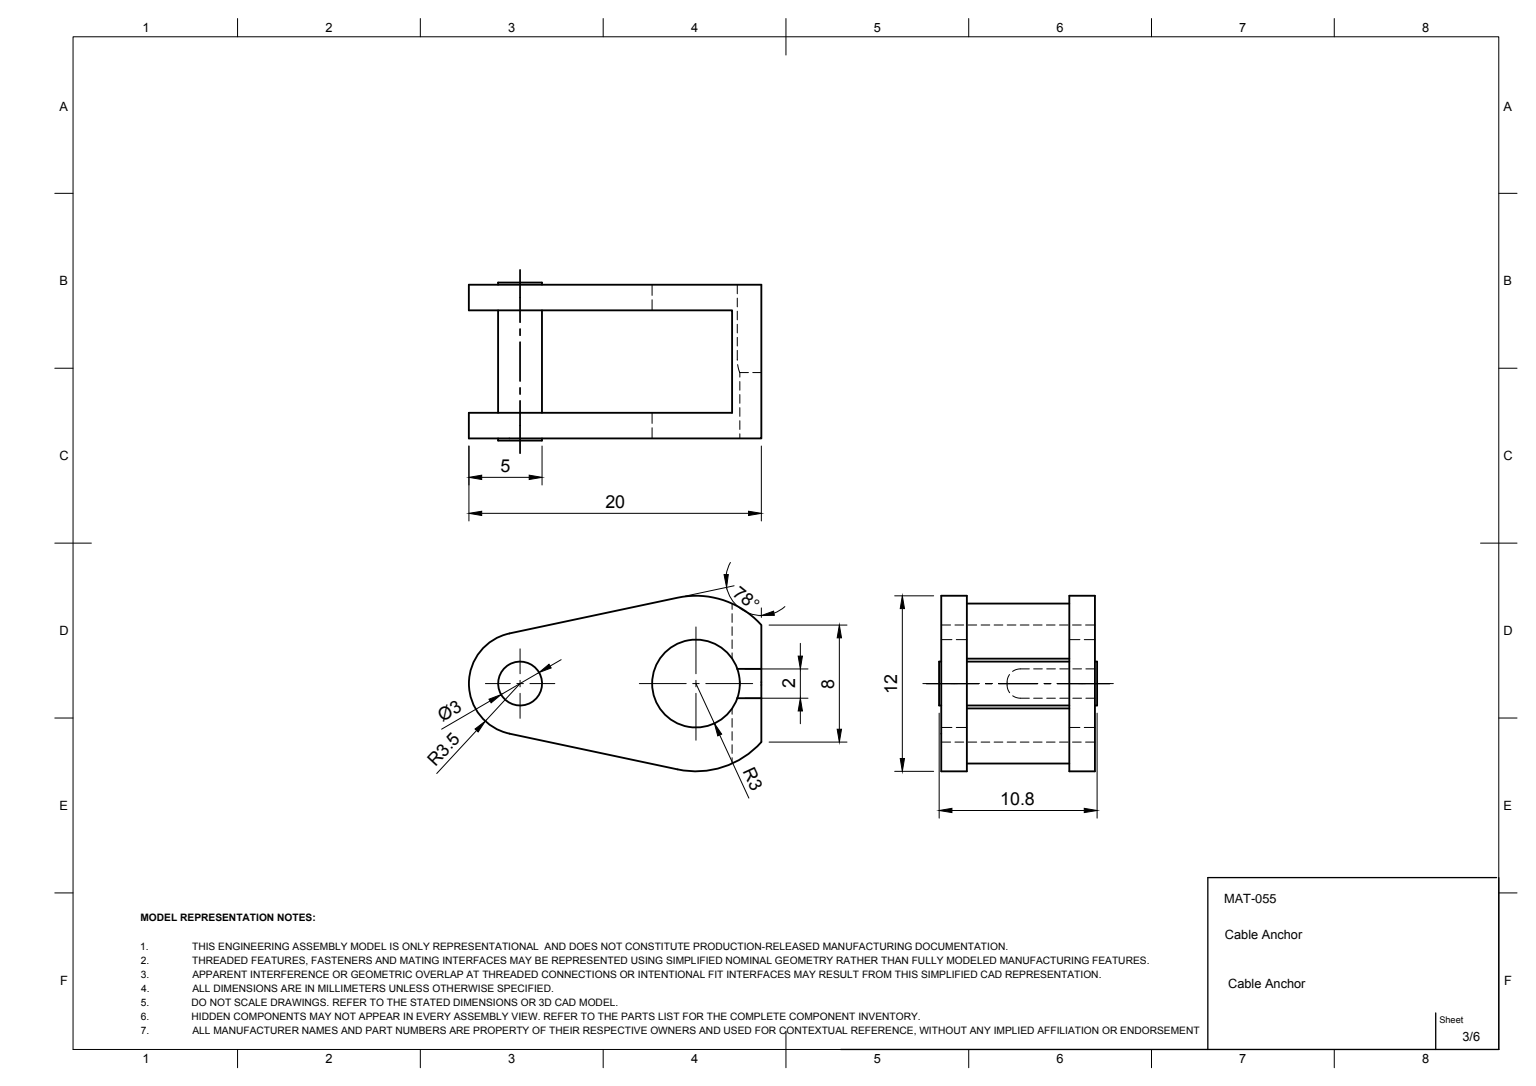
ISO-10303-21;
HEADER;
FILE_DESCRIPTION (('STEP AP214'),
    '1' );
FILE_NAME ('Cable Anchor.step',
    '2026-10-30T09:41:00',
    ( '' ),
    ( '' ),
    'SwSTEP 2.0',
    'SolidWorks 2020',
    '' );
FILE_SCHEMA (( 'AUTOMOTIVE_DESIGN' ));
ENDSEC;

DATA;
#81=ORIENTED_EDGE ( 'NONE', *, *, #25738, .F. ) ;
#83=CARTESIAN_POINT ( 'NONE',  ( 86.34560043013698305, -9.320000780048239619, -16.89321520033831447 ) ) ;
#175=AXIS2_PLACEMENT_3D ( 'NONE', #36006, #42871, #25989 ) ;
#203=EDGE_CURVE ( 'NONE', #36947, #44995, #9172, .T. ) ;
#218=CARTESIAN_POINT ( 'NONE',  ( 89.13600071704317429, -10.42165226880396567, -14.07015947738872796 ) ) ;
#224=LINE ( 'NONE', #17347, #39403 ) ;
#244=EDGE_LOOP ( 'NONE', ( #3351, #8690, #1510, #25931, #38519, #27404, #20407, #392, #9598, #8626 ) ) ;
#260=VECTOR ( 'NONE', #38746, 1000.000000000000000 ) ;
#392=ORIENTED_EDGE ( 'NONE', *, *, #6669, .F. ) ;
#446=CYLINDRICAL_SURFACE ( 'NONE', #37941, 1.499999999999996225 ) ;
#523=VERTEX_POINT ( 'NONE', #21002 ) ;
#586=LINE ( 'NONE', #7416, #43252 ) ;
#637=CARTESIAN_POINT ( 'NONE',  ( 77.25325688895158294, -4.012910213732562070, -16.89321520033831447 ) ) ;
#742=ORIENTED_EDGE ( 'NONE', *, *, #32280, .T. ) ;
#831=PRODUCT_DEFINITION_SHAPE ( 'NONE', 'NONE',  #16477 ) ;
#848=LINE ( 'NONE', #18639, #17728 ) ;
#855=DIRECTION ( 'NONE',  ( 0.000000000000000000, 0.000000000000000000, -1.000000000000000000 ) ) ;
#861=EDGE_CURVE ( 'NONE', #37401, #29422, #44018, .T. ) ;
#882=LINE ( 'NONE', #14801, #2318 ) ;
#1093=DIRECTION ( 'NONE',  ( 0.5040994586965589219, 0.8636456077245089347, 0.000000000000000000 ) ) ;
#1108=ORIENTED_EDGE ( 'NONE', *, *, #40951, .T. ) ;
#1150=DIRECTION ( 'NONE',  ( 0.5040994586965589219, 0.8636456077245089347, 0.000000000000000000 ) ) ;
#1340=CARTESIAN_POINT ( 'NONE',  ( 88.41031260927115909, -11.49916342651943957, -13.77494911842194369 ) ) ;
#1447=CARTESIAN_POINT ( 'NONE',  ( 83.75466360696344736, -7.807702403958562520, -8.143215200338314474 ) ) ;
#1510=ORIENTED_EDGE ( 'NONE', *, *, #22776, .F. ) ;
#1585=VECTOR ( 'NONE', #34649, 1000.000000000000000 ) ;
#1711=ORIENTED_EDGE ( 'NONE', *, *, #19855, .F. ) ;
#1718=CARTESIAN_POINT ( 'NONE',  ( 85.72471707980444933, -15.28778963902104060, -16.89321520033831447 ) ) ;
#1721=LINE ( 'NONE', #29548, #15713 ) ;
#1789=DIRECTION ( 'NONE',  ( 0.000000000000000000, 0.000000000000000000, 1.000000000000000000 ) ) ;
#1790=CARTESIAN_POINT ( 'NONE',  ( 82.31000308962319423, -13.76004065658516673, -8.143215200338314474 ) ) ;
#1794=CARTESIAN_POINT ( 'NONE',  ( 89.29245855188943892, -9.882163754870950001, -18.64321520033831803 ) ) ;
#1818=ORIENTED_EDGE ( 'NONE', *, *, #22126, .F. ) ;
#1835=CARTESIAN_POINT ( 'NONE',  ( 86.34560043013698305, -9.320000780048239619, -16.89321520033831447 ) ) ;
#1843=AXIS2_PLACEMENT_3D ( 'NONE', #8029, #11011, #28565 ) ;
#1857=PLANE ( 'NONE',  #19264 ) ;
#1947=DIRECTION ( 'NONE',  ( 0.6725995567522981000, 0.7400066460894877407, -0.000000000000000000 ) ) ;
#2013=EDGE_LOOP ( 'NONE', ( #16435, #12122, #81, #28622 ) ) ;
#2022=AXIS2_PLACEMENT_3D ( 'NONE', #28422, #15182, #21574 ) ;
#2037=EDGE_CURVE ( 'NONE', #38611, #14451, #22949, .T. ) ;
#2041=APPLICATION_CONTEXT ( 'automotive_design' ) ;
#2123=ORIENTED_EDGE ( 'NONE', *, *, #31988, .T. ) ;
#2144=DIRECTION ( 'NONE',  ( 0.8636456077245086016, -0.5040994586965593660, 0.000000000000000000 ) ) ;
#2184=EDGE_CURVE ( 'NONE', #38164, #19850, #25845, .T. ) ;
#2190=AXIS2_PLACEMENT_3D ( 'NONE', #12234, #8583, #22482 ) ;
#2195=VECTOR ( 'NONE', #28078, 1000.000000000000000 ) ;
#2318=VECTOR ( 'NONE', #7951, 1000.000000000000000 ) ;
#2389=DIRECTION ( 'NONE',  ( 0.000000000000000000, 0.000000000000000000, -1.000000000000000000 ) ) ;
#2435=CIRCLE ( 'NONE', #27952, 3.000000000000003997 ) ;
#2479=LINE ( 'NONE', #40116, #8942 ) ;
#2562=ORIENTED_EDGE ( 'NONE', *, *, #42601, .F. ) ;
#2639=PRODUCT_CONTEXT ( 'NONE', #2041, 'mechanical' ) ;
#2753=DIRECTION ( 'NONE',  ( -0.8636456077245080465, 0.5040994586965603652, 0.000000000000000000 ) ) ;
#2819=DIRECTION ( 'NONE',  ( 0.000000000000000000, 0.000000000000000000, 1.000000000000000000 ) ) ;
#2828=CARTESIAN_POINT ( 'NONE',  ( 89.70384154612264638, -12.43804770190545561, -13.24321520033830879 ) ) ;
#2894=ADVANCED_FACE ( 'NONE', ( #41375 ), #10569, .T. ) ;
#2910=ORIENTED_EDGE ( 'NONE', *, *, #16133, .T. ) ;
#2921=CIRCLE ( 'NONE', #20410, 1.499999999999996225 ) ;
#2971=CARTESIAN_POINT ( 'NONE',  ( 89.28655680551213436, -9.912712791071484730, -13.47323746212486562 ) ) ;
#2980=CYLINDRICAL_SURFACE ( 'NONE', #7519, 1.499999999999996225 ) ;
#2984=CIRCLE ( 'NONE', #11775, 3.000000000000003997 ) ;
#3002=ADVANCED_FACE ( 'NONE', ( #31747 ), #25144, .T. ) ;
#3083=CARTESIAN_POINT ( 'NONE',  ( 77.25325688895158294, -4.012910213732562070, -18.79321520033831661 ) ) ;
#3163=ORIENTED_EDGE ( 'NONE', *, *, #17306, .F. ) ;
#3280=VECTOR ( 'NONE', #28746, 1000.000000000000000 ) ;
#3313=EDGE_CURVE ( 'NONE', #6780, #34510, #28571, .T. ) ;
#3351=ORIENTED_EDGE ( 'NONE', *, *, #7188, .F. ) ;
#3382=EDGE_CURVE ( 'NONE', #44507, #41378, #20454, .T. ) ;
#3438=ORIENTED_EDGE ( 'NONE', *, *, #4563, .T. ) ;
#3451=( GEOMETRIC_REPRESENTATION_CONTEXT ( 3 ) GLOBAL_UNCERTAINTY_ASSIGNED_CONTEXT ( ( #12242 ) ) GLOBAL_UNIT_ASSIGNED_CONTEXT ( ( #15675, #12263, #22960 ) ) REPRESENTATION_CONTEXT ( 'NONE', 'WORKASPACE' ) );
#3489=ORIENTED_EDGE ( 'NONE', *, *, #37414, .F. ) ;
#3613=CIRCLE ( 'NONE', #9450, 3.500000000000003109 ) ;
#3624=DIRECTION ( 'NONE',  ( 0.000000000000000000, 0.000000000000000000, 1.000000000000000000 ) ) ;
#3636=CARTESIAN_POINT ( 'NONE',  ( 89.27431095563446206, -9.970335341274866536, -13.62791168839721578 ) ) ;
#3683=ORIENTED_EDGE ( 'NONE', *, *, #16133, .F. ) ;
#3709=CARTESIAN_POINT ( 'NONE',  ( 88.19154317003298615, -15.02898452507898241, -18.64321520033831803 ) ) ;
#3743=AXIS2_PLACEMENT_3D ( 'NONE', #39189, #18456, #14576 ) ;
#3804=CIRCLE ( 'NONE', #29297, 1.499999999999996225 ) ;
#3911=LINE ( 'NONE', #21701, #37404 ) ;
#3950=CIRCLE ( 'NONE', #25093, 0.8999999999999980238 ) ;
#3977=ORIENTED_EDGE ( 'NONE', *, *, #37659, .F. ) ;
#4067=ORIENTED_EDGE ( 'NONE', *, *, #25596, .F. ) ;
#4088=AXIS2_PLACEMENT_3D ( 'NONE', #23483, #22400, #18978 ) ;
#4120=EDGE_CURVE ( 'NONE', #19817, #22660, #18631, .T. ) ;
#4147=UNCERTAINTY_MEASURE_WITH_UNIT (LENGTH_MEASURE( 1.000000000000000082E-05 ), #7073, 'distance_accuracy_value', 'NONE');
#4169=DIRECTION ( 'NONE',  ( 0.8636456077245092677, -0.5040994586965584778, 0.000000000000000000 ) ) ;
#4190=CARTESIAN_POINT ( 'NONE',  ( 88.28425963449632263, -11.60945497031996787, -8.143215200338314474 ) ) ;
#4205=EDGE_LOOP ( 'NONE', ( #36138, #2910, #18407, #16763 ) ) ;
#4307=CARTESIAN_POINT ( 'NONE',  ( 88.75490232214124831, -11.10765887499229088, -14.11402746727662638 ) ) ;
#4405=EDGE_CURVE ( 'NONE', #18186, #38837, #25230, .T. ) ;
#4453=DIRECTION ( 'NONE',  ( 0.8636456077245080465, -0.5040994586965603652, 0.000000000000000000 ) ) ;
#4455=DIRECTION ( 'NONE',  ( 0.000000000000000000, 0.000000000000000000, -1.000000000000000000 ) ) ;
#4515=ADVANCED_FACE ( 'NONE', ( #12148, #37370, #42935 ), #9568, .T. ) ;
#4520=DIRECTION ( 'NONE',  ( 0.000000000000000000, 0.000000000000000000, 1.000000000000000000 ) ) ;
#4522=ORIENTED_EDGE ( 'NONE', *, *, #16161, .T. ) ;
#4545=DIRECTION ( 'NONE',  ( 0.000000000000000000, 0.000000000000000000, 1.000000000000000000 ) ) ;
#4557=LINE ( 'NONE', #21670, #3280 ) ;
#4563=EDGE_CURVE ( 'NONE', #41325, #5895, #29246, .T. ) ;
#4823=ADVANCED_FACE ( 'NONE', ( #25529 ), #25080, .F. ) ;
#4838=CARTESIAN_POINT ( 'NONE',  ( 88.98550738977573360, -10.74509419609185379, -14.14321520033831625 ) ) ;
#4842=DIRECTION ( 'NONE',  ( 0.5040994586965589219, 0.8636456077245089347, 0.000000000000000000 ) ) ;
#4981=LINE ( 'NONE', #22759, #37743 ) ;
#4992=ORIENTED_EDGE ( 'NONE', *, *, #41240, .T. ) ;
#5025=ADVANCED_FACE ( 'NONE', ( #22120 ), #12540, .T. ) ;
#5032=CARTESIAN_POINT ( 'NONE',  ( 77.05532149770296257, 0.06670422450934243574, -8.143215200338314474 ) ) ;
#5162=STYLED_ITEM ( 'NONE', ( #21425 ), #34112 ) ;
#5189=( GEOMETRIC_REPRESENTATION_CONTEXT ( 3 ) GLOBAL_UNCERTAINTY_ASSIGNED_CONTEXT ( ( #4147 ) ) GLOBAL_UNIT_ASSIGNED_CONTEXT ( ( #7073, #34041, #28503 ) ) REPRESENTATION_CONTEXT ( 'NONE', 'WORKASPACE' ) );
#5203=DIRECTION ( 'NONE',  ( -0.9495615000563050190, 0.3135808629537517600, 0.000000000000000000 ) ) ;
#5292=DIRECTION ( 'NONE',  ( 0.8636456077245089347, -0.5040994586965589219, 0.000000000000000000 ) ) ;
#5302=ORIENTED_EDGE ( 'NONE', *, *, #4120, .T. ) ;
#5305=FACE_OUTER_BOUND ( 'NONE', #20275, .T. ) ;
#5331=ORIENTED_EDGE ( 'NONE', *, *, #23077, .F. ) ;
#5350=CARTESIAN_POINT ( 'NONE',  ( 90.71204046351577688, -10.71075648645643774, -13.24321520033830879 ) ) ;
#5405=DIRECTION ( 'NONE',  ( -0.8636456077245088236, 0.5040994586965589219, 0.000000000000000000 ) ) ;
#5486=CARTESIAN_POINT ( 'NONE',  ( 90.15753105894957287, -11.66076665495339348, -14.14321520033831625 ) ) ;
#5565=AXIS2_PLACEMENT_3D ( 'NONE', #34275, #2819, #9907 ) ;
#5730=DIRECTION ( 'NONE',  ( 0.000000000000000000, 0.000000000000000000, 1.000000000000000000 ) ) ;
#5796=DIRECTION ( 'NONE',  ( 0.000000000000000000, 0.000000000000000000, 1.000000000000000000 ) ) ;
#5802=DIRECTION ( 'NONE',  ( 0.8636456077245088236, -0.5040994586965589219, 0.000000000000000000 ) ) ;
#5826=ORIENTED_EDGE ( 'NONE', *, *, #25693, .T. ) ;
#5875=AXIS2_PLACEMENT_3D ( 'NONE', #16189, #26219, #12545 ) ;
#5895=VERTEX_POINT ( 'NONE', #39164 ) ;
#5937=DIRECTION ( 'NONE',  ( 0.8636456077245086016, -0.5040994586965593660, 0.000000000000000000 ) ) ;
#5991=EDGE_LOOP ( 'NONE', ( #15098, #6340 ) ) ;
#5994=VECTOR ( 'NONE', #14852, 1000.000000000000000 ) ;
#6040=CARTESIAN_POINT ( 'NONE',  ( 82.31000308962319423, -13.76004065658516673, -16.89321520033831447 ) ) ;
#6046=CARTESIAN_POINT ( 'NONE',  ( 88.22708560785949317, -3.622631779710408395, -8.143215200338314474 ) ) ;
#6057=AXIS2_PLACEMENT_3D ( 'NONE', #16541, #16310, #39793 ) ;
#6075=ADVANCED_FACE ( 'NONE', ( #29804 ), #12487, .T. ) ;
#6132=MANIFOLD_SOLID_BREP ( 'NONE', #43263 ) ;
#6139=DIRECTION ( 'NONE',  ( 0.8636456077245080465, -0.5040994586965603652, 0.000000000000000000 ) ) ;
#6163=ORIENTED_EDGE ( 'NONE', *, *, #26420, .T. ) ;
#6170=CARTESIAN_POINT ( 'NONE',  ( 89.25356269854076174, -10.05861921418335392, -13.77344656902741526 ) ) ;
#6179=CARTESIAN_POINT ( 'NONE',  ( 75.95778847736481509, -3.256761025687722189, -7.993215200338315007 ) ) ;
#6247=VECTOR ( 'NONE', #6312, 1000.000000000000000 ) ;
#6258=VECTOR ( 'NONE', #12751, 1000.000000000000000 ) ;
#6312=DIRECTION ( 'NONE',  ( 0.000000000000000000, 0.000000000000000000, -1.000000000000000000 ) ) ;
#6337=CIRCLE ( 'NONE', #44918, 1.499999999999996225 ) ;
#6340=ORIENTED_EDGE ( 'NONE', *, *, #30362, .F. ) ;
#6369=EDGE_LOOP ( 'NONE', ( #33977, #18603, #8506, #6643 ) ) ;
#6438=AXIS2_PLACEMENT_3D ( 'NONE', #41953, #35762, #10718 ) ;
#6493=ORIENTED_EDGE ( 'NONE', *, *, #18626, .T. ) ;
#6547=DIRECTION ( 'NONE',  ( 0.000000000000000000, 0.000000000000000000, 1.000000000000000000 ) ) ;
#6609=ORIENTED_EDGE ( 'NONE', *, *, #44531, .T. ) ;
#6630=CYLINDRICAL_SURFACE ( 'NONE', #41605, 5.999999999999997335 ) ;
#6643=ORIENTED_EDGE ( 'NONE', *, *, #32613, .F. ) ;
#6658=DIRECTION ( 'NONE',  ( 0.000000000000000000, 0.000000000000000000, -1.000000000000000000 ) ) ;
#6669=EDGE_CURVE ( 'NONE', #43343, #14177, #24580, .T. ) ;
#6688=LINE ( 'NONE', #44996, #33195 ) ;
#6720=VERTEX_POINT ( 'NONE', #39790 ) ;
#6780=VERTEX_POINT ( 'NONE', #26109 ) ;
#6800=ORIENTED_EDGE ( 'NONE', *, *, #32283, .T. ) ;
#6851=CARTESIAN_POINT ( 'NONE',  ( 89.21236786697126320, -10.20601085363140648, -13.93603761494362736 ) ) ;
#6862=CARTESIAN_POINT ( 'NONE',  ( 88.93653725331050452, -10.83229915613791761, -18.64321520033831803 ) ) ;
#6883=CARTESIAN_POINT ( 'NONE',  ( 75.95778847736481509, -3.256761025687722189, -18.64321520033831803 ) ) ;
#6885=ADVANCED_FACE ( 'NONE', ( #29752 ), #40247, .T. ) ;
#6924=EDGE_LOOP ( 'NONE', ( #28323, #7052, #35262, #3977 ) ) ;
#7007=CARTESIAN_POINT ( 'NONE',  ( 82.31000308962319423, -13.76004065658516673, -16.89321520033831447 ) ) ;
#7019=CARTESIAN_POINT ( 'NONE',  ( 86.34560043013698305, -9.320000780048239619, -14.14321520033831625 ) ) ;
#7052=ORIENTED_EDGE ( 'NONE', *, *, #42339, .T. ) ;
#7066=CARTESIAN_POINT ( 'NONE',  ( 89.29245855188943892, -9.882163754870950001, -13.24321520033830879 ) ) ;
#7073=( LENGTH_UNIT ( ) NAMED_UNIT ( * ) SI_UNIT ( .MILLI., .METRE. ) );
#7091=STYLED_ITEM('',(#45169),#6132);
#7142=ORIENTED_EDGE ( 'NONE', *, *, #15130, .T. ) ;
#7188=EDGE_CURVE ( 'NONE', #33083, #44381, #23615, .T. ) ;
#7209=ORIENTED_EDGE ( 'NONE', *, *, #24743, .F. ) ;
#7329=LINE ( 'NONE', #21248, #32135 ) ;
#7416=CARTESIAN_POINT ( 'NONE',  ( 88.19154317003298615, -15.02898452507898241, -18.64321520033831803 ) ) ;
#7484=CARTESIAN_POINT ( 'NONE',  ( 88.28425963449632263, -11.60945497031996787, -13.24321520033830879 ) ) ;
#7503=CARTESIAN_POINT ( 'NONE',  ( 85.83930302032700865, -9.140269361470602760, -13.24321520033831412 ) ) ;
#7519=AXIS2_PLACEMENT_3D ( 'NONE', #6179, #16908, #2753 ) ;
#7547=DIRECTION ( 'NONE',  ( 0.000000000000000000, 0.000000000000000000, 1.000000000000000000 ) ) ;
#7566=CIRCLE ( 'NONE', #44729, 1.499999999999996225 ) ;
#7645=CARTESIAN_POINT ( 'NONE',  ( 89.33740294208338639, -9.098375579515472822, -16.89321520033831447 ) ) ;
#7681=AXIS2_PLACEMENT_3D ( 'NONE', #38357, #10131, #14205 ) ;
#7730=EDGE_CURVE ( 'NONE', #13487, #34510, #18139, .T. ) ;
#7736=CARTESIAN_POINT ( 'NONE',  ( 88.77226126511364157, -11.08399544887646293, -14.12116704279862667 ) ) ;
#7738=FACE_OUTER_BOUND ( 'NONE', #26887, .T. ) ;
#7766=AXIS2_PLACEMENT_3D ( 'NONE', #29770, #1947, #36150 ) ;
#7781=CARTESIAN_POINT ( 'NONE',  ( 75.95778847736481509, -3.256761025687722189, -16.89321520033831447 ) ) ;
#7819=ORIENTED_EDGE ( 'NONE', *, *, #2184, .F. ) ;
#7951=DIRECTION ( 'NONE',  ( 0.000000000000000000, 0.000000000000000000, 1.000000000000000000 ) ) ;
#7961=CARTESIAN_POINT ( 'NONE',  ( 88.28425963449630842, -11.60945497031996787, -13.33030055912934486 ) ) ;
#7973=FACE_OUTER_BOUND ( 'NONE', #19915, .T. ) ;
#7979=DIRECTION ( 'NONE',  ( -0.8636456077245080465, 0.5040994586965603652, 0.000000000000000000 ) ) ;
#8029=CARTESIAN_POINT ( 'NONE',  ( 75.95778847736481509, -3.256761025687722189, -7.993215200338315007 ) ) ;
#8095=ORIENTED_EDGE ( 'NONE', *, *, #37552, .T. ) ;
#8179=DIRECTION ( 'NONE',  ( 0.000000000000000000, 0.000000000000000000, 1.000000000000000000 ) ) ;
#8204=VERTEX_POINT ( 'NONE', #14455 ) ;
#8238=CARTESIAN_POINT ( 'NONE',  ( 75.95778847736481509, -3.256761025687722189, -18.64321520033831803 ) ) ;
#8336=DIRECTION ( 'NONE',  ( -0.8636456077245080465, 0.5040994586965603652, 0.000000000000000000 ) ) ;
#8380=ORIENTED_EDGE ( 'NONE', *, *, #12193, .F. ) ;
#8407=FACE_OUTER_BOUND ( 'NONE', #24964, .T. ) ;
#8426=AXIS2_PLACEMENT_3D ( 'NONE', #24813, #21391, #28693 ) ;
#8434=CARTESIAN_POINT ( 'NONE',  ( 75.95778847736481509, -3.256761025687722189, -7.993215200338315007 ) ) ;
#8452=DIRECTION ( 'NONE',  ( -0.8636456077245089347, 0.5040994586965589219, 0.000000000000000000 ) ) ;
#8506=ORIENTED_EDGE ( 'NONE', *, *, #7730, .F. ) ;
#8562=EDGE_CURVE ( 'NONE', #18186, #10189, #15022, .T. ) ;
#8583=DIRECTION ( 'NONE',  ( 0.000000000000000000, 0.000000000000000000, 1.000000000000000000 ) ) ;
#8626=ORIENTED_EDGE ( 'NONE', *, *, #35895, .F. ) ;
#8634=ORIENTED_EDGE ( 'NONE', *, *, #27571, .F. ) ;
#8643=CARTESIAN_POINT ( 'NONE',  ( 88.58241854558018247, -11.31884705245859735, -13.99297490352741846 ) ) ;
#8690=ORIENTED_EDGE ( 'NONE', *, *, #20333, .F. ) ;
#8715=FACE_BOUND ( 'NONE', #13443, .T. ) ;
#8802=DIRECTION ( 'NONE',  ( 0.000000000000000000, 0.000000000000000000, 1.000000000000000000 ) ) ;
#8833=ADVANCED_FACE ( 'NONE', ( #8407 ), #22984, .T. ) ;
#8836=AXIS2_PLACEMENT_3D ( 'NONE', #8238, #39244, #26240 ) ;
#8851=CARTESIAN_POINT ( 'NONE',  ( 86.34560043013698305, -9.320000780048239619, -18.64321520033831803 ) ) ;
#8869=CARTESIAN_POINT ( 'NONE',  ( 88.22708560785949317, -3.622631779710408395, -18.64321520033831803 ) ) ;
#8881=DIRECTION ( 'NONE',  ( 0.000000000000000000, 0.000000000000000000, -1.000000000000000000 ) ) ;
#8887=ADVANCED_FACE ( 'NONE', ( #42849 ), #18224, .F. ) ;
#8893=CARTESIAN_POINT ( 'NONE',  ( 86.84969988883354119, -8.456355172323730685, -8.143215200338314474 ) ) ;
#8920=DIRECTION ( 'NONE',  ( 0.000000000000000000, 0.000000000000000000, 1.000000000000000000 ) ) ;
#8941=EDGE_LOOP ( 'NONE', ( #5331, #1108, #28713, #36956 ) ) ;
#8942=VECTOR ( 'NONE', #36676, 1000.000000000000000 ) ;
#9032=EDGE_CURVE ( 'NONE', #9608, #38611, #4981, .T. ) ;
#9080=DIRECTION ( 'NONE',  ( 0.000000000000000000, 0.000000000000000000, 1.000000000000000000 ) ) ;
#9119=LINE ( 'NONE', #8893, #43025 ) ;
#9130=ADVANCED_FACE ( 'NONE', ( #18893 ), #15249, .F. ) ;
#9138=DIRECTION ( 'NONE',  ( 0.7400066460894876297, -0.6725995567522979890, -0.000000000000000000 ) ) ;
#9172=LINE ( 'NONE', #12829, #22849 ) ;
#9331=EDGE_LOOP ( 'NONE', ( #22443, #42916, #24039, #4522, #19586, #21662, #25451, #16566, #28743 ) ) ;
#9358=AXIS2_PLACEMENT_3D ( 'NONE', #8851, #8179, #43741 ) ;
#9422=DIRECTION ( 'NONE',  ( 0.5040994586965589219, 0.8636456077245088236, 0.000000000000000000 ) ) ;
#9450=AXIS2_PLACEMENT_3D ( 'NONE', #6883, #42215, #38324 ) ;
#9458=ORIENTED_EDGE ( 'NONE', *, *, #7188, .T. ) ;
#9503=CARTESIAN_POINT ( 'NONE',  ( 75.95778847736481509, -3.256761025687722189, -18.79321520033831661 ) ) ;
#9568=PLANE ( 'NONE',  #33211 ) ;
#9587=CIRCLE ( 'NONE', #3743, 1.499999999999996225 ) ;
#9590=EDGE_LOOP ( 'NONE', ( #9737, #20621, #9848, #29851, #3163, #31551, #40147, #7819 ) ) ;
#9598=ORIENTED_EDGE ( 'NONE', *, *, #34790, .F. ) ;
#9602=EDGE_CURVE ( 'NONE', #9608, #18186, #28225, .T. ) ;
#9608=VERTEX_POINT ( 'NONE', #21595 ) ;
#9731=EDGE_CURVE ( 'NONE', #36064, #37401, #18138, .T. ) ;
#9737=ORIENTED_EDGE ( 'NONE', *, *, #10396, .F. ) ;
#9764=AXIS2_PLACEMENT_3D ( 'NONE', #9503, #40290, #33196 ) ;
#9838=DIRECTION ( 'NONE',  ( 0.000000000000000000, 0.000000000000000000, -1.000000000000000000 ) ) ;
#9848=ORIENTED_EDGE ( 'NONE', *, *, #9032, .T. ) ;
#9886=VECTOR ( 'NONE', #42926, 1000.000000000000000 ) ;
#9906=VERTEX_POINT ( 'NONE', #32518 ) ;
#9907=DIRECTION ( 'NONE',  ( 0.8636456077245080465, -0.5040994586965603652, 0.000000000000000000 ) ) ;
#9940=CARTESIAN_POINT ( 'NONE',  ( 83.75466360696344736, -7.807702403958562520, -16.89321520033831447 ) ) ;
#9968=CARTESIAN_POINT ( 'NONE',  ( 89.70384154612264638, -12.43804770190545561, -8.143215200338314474 ) ) ;
#9986=DIRECTION ( 'NONE',  ( 0.000000000000000000, 0.000000000000000000, -1.000000000000000000 ) ) ;
#10061=CARTESIAN_POINT ( 'NONE',  ( 89.29245855188943892, -9.882163754870950001, -13.29917559099935254 ) ) ;
#10131=DIRECTION ( 'NONE',  ( -0.8636456077245089347, 0.5040994586965589219, 0.000000000000000000 ) ) ;
#10134=EDGE_LOOP ( 'NONE', ( #6800, #43372, #6609, #23190, #35517, #2123, #32085, #34222, #10402, #35572, #13202 ) ) ;
#10189=VERTEX_POINT ( 'NONE', #5032 ) ;
#10251=CARTESIAN_POINT ( 'NONE',  ( 86.34560043013698305, -9.320000780048239619, -14.14321520033831625 ) ) ;
#10352=VECTOR ( 'NONE', #4520, 1000.000000000000000 ) ;
#10396=EDGE_CURVE ( 'NONE', #12781, #38164, #21537, .T. ) ;
#10402=ORIENTED_EDGE ( 'NONE', *, *, #26420, .F. ) ;
#10414=DIRECTION ( 'NONE',  ( -0.9495615000563050190, 0.3135808629537517600, 0.000000000000000000 ) ) ;
#10439=DIRECTION ( 'NONE',  ( 0.000000000000000000, 0.000000000000000000, -1.000000000000000000 ) ) ;
#10447=VERTEX_POINT ( 'NONE', #5486 ) ;
#10498=CARTESIAN_POINT ( 'NONE',  ( 89.27917506468355668, -9.947819920281929740, -13.57505156349929720 ) ) ;
#10567=AXIS2_PLACEMENT_3D ( 'NONE', #26792, #5796, #2144 ) ;
#10569=PLANE ( 'NONE',  #7681 ) ;
#10696=FACE_OUTER_BOUND ( 'NONE', #32936, .T. ) ;
#10715=DIRECTION ( 'NONE',  ( 0.000000000000000000, 0.000000000000000000, 1.000000000000000000 ) ) ;
#10718=DIRECTION ( 'NONE',  ( 0.5040994586965589219, 0.8636456077245089347, 0.000000000000000000 ) ) ;
#10726=DIRECTION ( 'NONE',  ( 0.8636456077245086016, -0.5040994586965593660, 0.000000000000000000 ) ) ;
#10727=DIRECTION ( 'NONE',  ( 1.000000000000000000, 0.000000000000000000, 0.000000000000000000 ) ) ;
#10840=EDGE_CURVE ( 'NONE', #19108, #33768, #3613, .T. ) ;
#10896=AXIS2_PLACEMENT_3D ( 'NONE', #12166, #15581, #32446 ) ;
#10947=CARTESIAN_POINT ( 'NONE',  ( 74.66232006577804725, -2.500611837642884527, -8.143215200338314474 ) ) ;
#10999=VERTEX_POINT ( 'NONE', #42886 ) ;
#11011=DIRECTION ( 'NONE',  ( 0.000000000000000000, 0.000000000000000000, -1.000000000000000000 ) ) ;
#11074=ADVANCED_FACE ( 'NONE', ( #39230 ), #43106, .T. ) ;
#11080=EDGE_CURVE ( 'NONE', #19235, #8204, #40046, .T. ) ;
#11169=CARTESIAN_POINT ( 'NONE',  ( 88.69904943327698277, -11.18046741462036842, -14.08431115565796254 ) ) ;
#11242=CARTESIAN_POINT ( 'NONE',  ( 77.25325688895158294, -4.012910213732562070, -7.993215200338315007 ) ) ;
#11347=AXIS2_PLACEMENT_3D ( 'NONE', #29769, #43679, #27036 ) ;
#11355=CARTESIAN_POINT ( 'NONE',  ( 86.34560043013698305, -9.320000780048239619, -8.143215200338314474 ) ) ;
#11382=ORIENTED_EDGE ( 'NONE', *, *, #203, .F. ) ;
#11436=CARTESIAN_POINT ( 'NONE',  ( 77.05532149770296257, 0.06670422450934243574, -9.893215200338316251 ) ) ;
#11437=CARTESIAN_POINT ( 'NONE',  ( 85.45605303719084134, -15.74807682313488222, -9.893215200338316251 ) ) ;
#11613=CARTESIAN_POINT ( 'NONE',  ( 88.63266681459825236, -11.26170729784157665, -14.03921856447226446 ) ) ;
#11689=ORIENTED_EDGE ( 'NONE', *, *, #24861, .F. ) ;
#11775=AXIS2_PLACEMENT_3D ( 'NONE', #20245, #9986, #45083 ) ;
#11821=LINE ( 'NONE', #28927, #10352 ) ;
#11840=CIRCLE ( 'NONE', #175, 3.000000000000003997 ) ;
#11847=DIRECTION ( 'NONE',  ( 0.8636456077245086016, -0.5040994586965593660, 0.000000000000000000 ) ) ;
#11993=LINE ( 'NONE', #16316, #21692 ) ;
#12083=AXIS2_PLACEMENT_3D ( 'NONE', #20400, #13554, #41385 ) ;
#12097=CIRCLE ( 'NONE', #25929, 1.499999999999996225 ) ;
#12105=EDGE_LOOP ( 'NONE', ( #18265, #25083, #40561, #43336 ) ) ;
#12122=ORIENTED_EDGE ( 'NONE', *, *, #40151, .F. ) ;
#12148=FACE_BOUND ( 'NONE', #5991, .T. ) ;
#12166=CARTESIAN_POINT ( 'NONE',  ( 75.95778847736481509, -3.256761025687722189, -18.79321520033831661 ) ) ;
#12193=EDGE_CURVE ( 'NONE', #43318, #38775, #21881, .T. ) ;
#12234=CARTESIAN_POINT ( 'NONE',  ( 86.34560043013698305, -9.320000780048239619, -16.89321520033831447 ) ) ;
#12242=UNCERTAINTY_MEASURE_WITH_UNIT (LENGTH_MEASURE( 1.000000000000000082E-05 ), #15675, 'distance_accuracy_value', 'NONE');
#12263=( NAMED_UNIT ( * ) PLANE_ANGLE_UNIT ( ) SI_UNIT ( $, .RADIAN. ) );
#12316=CARTESIAN_POINT ( 'NONE',  ( 90.20794100481921873, -11.57440209418094668, -18.64321520033831803 ) ) ;
#12320=PLANE ( 'NONE',  #5875 ) ;
#12375=AXIS2_PLACEMENT_3D ( 'NONE', #42185, #21649, #10727 ) ;
#12402=CARTESIAN_POINT ( 'NONE',  ( 75.95778847736481509, -3.256761025687722189, -18.64321520033831803 ) ) ;
#12482=LINE ( 'NONE', #36624, #14022 ) ;
#12487=CYLINDRICAL_SURFACE ( 'NONE', #14321, 1.499999999999996225 ) ;
#12540=PLANE ( 'NONE',  #21578 ) ;
#12545=DIRECTION ( 'NONE',  ( 0.5040994586965589219, 0.8636456077245089347, 0.000000000000000000 ) ) ;
#12546=VECTOR ( 'NONE', #23783, 1000.000000000000114 ) ;
#12635=LINE ( 'NONE', #26982, #37653 ) ;
#12641=DIRECTION ( 'NONE',  ( -0.7400066460894876297, 0.6725995567522979890, 0.000000000000000000 ) ) ;
#12731=AXIS2_PLACEMENT_3D ( 'NONE', #36959, #5730, #19650 ) ;
#12736=ORIENTED_EDGE ( 'NONE', *, *, #42339, .F. ) ;
#12751=DIRECTION ( 'NONE',  ( 0.000000000000000000, 0.000000000000000000, 1.000000000000000000 ) ) ;
#12781=VERTEX_POINT ( 'NONE', #42500 ) ;
#12829=CARTESIAN_POINT ( 'NONE',  ( 82.31000308962319423, -13.76004065658516673, -18.64321520033831803 ) ) ;
#12900=DIRECTION ( 'NONE',  ( -0.5040994586965557023, -0.8636456077245108220, 0.000000000000000000 ) ) ;
#13202=ORIENTED_EDGE ( 'NONE', *, *, #15130, .F. ) ;
#13214=ORIENTED_EDGE ( 'NONE', *, *, #22126, .T. ) ;
#13313=( NAMED_UNIT ( * ) PLANE_ANGLE_UNIT ( ) SI_UNIT ( $, .RADIAN. ) );
#13338=CIRCLE ( 'NONE', #40278, 5.999999999999997335 ) ;
#13361=CARTESIAN_POINT ( 'NONE',  ( 85.94012291206632881, -8.967540239925700263, -13.24321520033831412 ) ) ;
#13376=ADVANCED_FACE ( 'NONE', ( #43740 ), #25958, .T. ) ;
#13392=CARTESIAN_POINT ( 'NONE',  ( 83.75466360696344736, -7.807702403958562520, -18.64321520033831803 ) ) ;
#13443=EDGE_LOOP ( 'NONE', ( #32627, #38198 ) ) ;
#13487=VERTEX_POINT ( 'NONE', #42840 ) ;
#13506=CARTESIAN_POINT ( 'NONE',  ( 91.23658249893594530, -5.844616714554617509, -16.89321520033831447 ) ) ;
#13554=DIRECTION ( 'NONE',  ( 0.000000000000000000, 0.000000000000000000, -1.000000000000000000 ) ) ;
#13634=CARTESIAN_POINT ( 'NONE',  ( 89.33740294208338639, -9.098375579515472822, -18.64321520033831803 ) ) ;
#13690=ORIENTED_EDGE ( 'NONE', *, *, #4405, .T. ) ;
#13802=CYLINDRICAL_SURFACE ( 'NONE', #44856, 0.8999999999999980238 ) ;
#13891=VECTOR ( 'NONE', #20205, 1000.000000000000114 ) ;
#14004=ORIENTED_EDGE ( 'NONE', *, *, #11080, .F. ) ;
#14022=VECTOR ( 'NONE', #40292, 1000.000000000000000 ) ;
#14051=EDGE_CURVE ( 'NONE', #22660, #19817, #9587, .T. ) ;
#14058=CARTESIAN_POINT ( 'NONE',  ( 90.25835095068887881, -11.48803753340849632, -13.24321520033831412 ) ) ;
#14109=CIRCLE ( 'NONE', #9764, 1.499999999999996225 ) ;
#14131=CARTESIAN_POINT ( 'NONE',  ( 89.13407410398241382, -10.42653939434942245, -14.07237609319362193 ) ) ;
#14138=( LENGTH_UNIT ( ) NAMED_UNIT ( * ) SI_UNIT ( .MILLI., .METRE. ) );
#14148=ORIENTED_EDGE ( 'NONE', *, *, #12193, .T. ) ;
#14177=VERTEX_POINT ( 'NONE', #5350 ) ;
#14205=DIRECTION ( 'NONE',  ( 0.5040994586965589219, 0.8636456077245089347, 0.000000000000000000 ) ) ;
#14321=AXIS2_PLACEMENT_3D ( 'NONE', #29128, #36628, #32755 ) ;
#14362=DIRECTION ( 'NONE',  ( -0.8636456077245080465, 0.5040994586965603652, 0.000000000000000000 ) ) ;
#14386=CARTESIAN_POINT ( 'NONE',  ( 88.22708560785949317, -3.622631779710408395, -8.143215200338314474 ) ) ;
#14451=VERTEX_POINT ( 'NONE', #44799 ) ;
#14455=CARTESIAN_POINT ( 'NONE',  ( 83.75466360696344736, -7.807702403958562520, -9.893215200338316251 ) ) ;
#14576=DIRECTION ( 'NONE',  ( -0.8636456077245080465, 0.5040994586965603652, 0.000000000000000000 ) ) ;
#14585=FILL_AREA_STYLE_COLOUR ( '', #16014 ) ;
#14588=DIRECTION ( 'NONE',  ( -0.5040994586965589219, -0.8636456077245089347, 0.000000000000000000 ) ) ;
#14605=AXIS2_PLACEMENT_3D ( 'NONE', #20347, #6658, #20568 ) ;
#14643=VECTOR ( 'NONE', #43327, 1000.000000000000114 ) ;
#14698=DIRECTION ( 'NONE',  ( 0.000000000000000000, 0.000000000000000000, -1.000000000000000000 ) ) ;
#14712=EDGE_CURVE ( 'NONE', #15181, #32644, #43243, .T. ) ;
#14801=CARTESIAN_POINT ( 'NONE',  ( 82.31000308962319423, -13.76004065658516673, -18.64321520033831803 ) ) ;
#14850=ORIENTED_EDGE ( 'NONE', *, *, #2037, .F. ) ;
#14852=DIRECTION ( 'NONE',  ( 0.5040994586965589219, 0.8636456077245088236, 0.000000000000000000 ) ) ;
#14860=DIRECTION ( 'NONE',  ( 0.8636456077245088236, -0.5040994586965589219, 0.000000000000000000 ) ) ;
#14905=DIRECTION ( 'NONE',  ( 0.5040994586965589219, 0.8636456077245088236, 0.000000000000000000 ) ) ;
#14979=VERTEX_POINT ( 'NONE', #22831 ) ;
#15022=LINE ( 'NONE', #38953, #15179 ) ;
#15033=VERTEX_POINT ( 'NONE', #27617 ) ;
#15035=CARTESIAN_POINT ( 'NONE',  ( 88.85502916797432249, -10.96495313371121050, -14.14321520033831625 ) ) ;
#15098=ORIENTED_EDGE ( 'NONE', *, *, #32283, .F. ) ;
#15130=EDGE_CURVE ( 'NONE', #34894, #37401, #38748, .T. ) ;
#15178=EDGE_CURVE ( 'NONE', #16620, #15181, #31463, .T. ) ;
#15179=VECTOR ( 'NONE', #3624, 1000.000000000000000 ) ;
#15181=VERTEX_POINT ( 'NONE', #31022 ) ;
#15182=DIRECTION ( 'NONE',  ( 0.000000000000000000, 0.000000000000000000, -1.000000000000000000 ) ) ;
#15214=DIRECTION ( 'NONE',  ( 0.8636456077245088236, -0.5040994586965589219, 0.000000000000000000 ) ) ;
#15249=PLANE ( 'NONE',  #18080 ) ;
#15254=CARTESIAN_POINT ( 'NONE',  ( 88.35915213937708756, -11.54718831182111849, -13.65586429604254626 ) ) ;
#15324=FACE_OUTER_BOUND ( 'NONE', #29838, .T. ) ;
#15325=ADVANCED_FACE ( 'NONE', ( #7973 ), #18906, .F. ) ;
#15363=MECHANICAL_DESIGN_GEOMETRIC_PRESENTATION_REPRESENTATION('',(#5162),#5189);
#15383=ORIENTED_EDGE ( 'NONE', *, *, #43156, .T. ) ;
#15402=CARTESIAN_POINT ( 'NONE',  ( 75.95778847736481509, -3.256761025687722189, -7.993215200338315007 ) ) ;
#15505=CARTESIAN_POINT ( 'NONE',  ( 82.31000308962319423, -13.76004065658516673, -18.64321520033831803 ) ) ;
#15517=LINE ( 'NONE', #11437, #5994 ) ;
#15558=AXIS2_PLACEMENT_3D ( 'NONE', #7503, #22045, #35938 ) ;
#15559=CARTESIAN_POINT ( 'NONE',  ( 86.34560043013698305, -9.320000780048239619, -18.64321520033831803 ) ) ;
#15581=DIRECTION ( 'NONE',  ( 0.000000000000000000, 0.000000000000000000, -1.000000000000000000 ) ) ;
#15590=DIRECTION ( 'NONE',  ( 0.000000000000000000, 0.000000000000000000, -1.000000000000000000 ) ) ;
#15628=ADVANCED_FACE ( 'NONE', ( #5305 ), #34018, .F. ) ;
#15635=CARTESIAN_POINT ( 'NONE',  ( 89.29245855188943892, -9.882163754870950001, -13.24321520033830879 ) ) ;
#15643=DIRECTION ( 'NONE',  ( 0.000000000000000000, 0.000000000000000000, 1.000000000000000000 ) ) ;
#15675=( LENGTH_UNIT ( ) NAMED_UNIT ( * ) SI_UNIT ( .MILLI., .METRE. ) );
#15713=VECTOR ( 'NONE', #15643, 1000.000000000000000 ) ;
#15742=DIRECTION ( 'NONE',  ( 0.8636456077245092677, -0.5040994586965584778, 0.000000000000000000 ) ) ;
#15788=DIRECTION ( 'NONE',  ( 0.000000000000000000, 0.000000000000000000, 1.000000000000000000 ) ) ;
#15789=DIRECTION ( 'NONE',  ( 0.000000000000000000, 0.000000000000000000, -1.000000000000000000 ) ) ;
#15908=EDGE_CURVE ( 'NONE', #19850, #27673, #31491, .T. ) ;
#16014=COLOUR_RGB ( '',0.7921568627450980005, 0.8196078431372548767, 0.9333333333333333481 ) ;
#16039=EDGE_LOOP ( 'NONE', ( #17861, #23908 ) ) ;
#16105=EDGE_CURVE ( 'NONE', #37436, #5895, #3804, .T. ) ;
#16133=EDGE_CURVE ( 'NONE', #18524, #32644, #15517, .T. ) ;
#16161=EDGE_CURVE ( 'NONE', #17596, #16972, #17486, .T. ) ;
#16189=CARTESIAN_POINT ( 'NONE',  ( 75.95778847736481509, -3.256761025687722189, -18.79321520033831661 ) ) ;
#16310=DIRECTION ( 'NONE',  ( 0.000000000000000000, 0.000000000000000000, -1.000000000000000000 ) ) ;
#16316=CARTESIAN_POINT ( 'NONE',  ( 77.25325688895158294, -4.012910213732562070, -7.993215200338315007 ) ) ;
#16353=CARTESIAN_POINT ( 'NONE',  ( 74.66232006577804725, -2.500611837642884527, -7.993215200338315007 ) ) ;
#16354=LINE ( 'NONE', #44182, #39106 ) ;
#16435=ORIENTED_EDGE ( 'NONE', *, *, #10396, .T. ) ;
#16477=PRODUCT_DEFINITION ( 'UNKNOWN', '', #20609, #37918 ) ;
#16481=VECTOR ( 'NONE', #15789, 1000.000000000000000 ) ;
#16541=CARTESIAN_POINT ( 'NONE',  ( 86.34560043013698305, -9.320000780048239619, -8.143215200338314474 ) ) ;
#16566=ORIENTED_EDGE ( 'NONE', *, *, #28388, .F. ) ;
#16620=VERTEX_POINT ( 'NONE', #1718 ) ;
#16681=EDGE_CURVE ( 'NONE', #6720, #26554, #13338, .T. ) ;
#16763=ORIENTED_EDGE ( 'NONE', *, *, #15178, .F. ) ;
#16794=ORIENTED_EDGE ( 'NONE', *, *, #20447, .T. ) ;
#16900=ORIENTED_EDGE ( 'NONE', *, *, #25693, .F. ) ;
#16908=DIRECTION ( 'NONE',  ( 0.000000000000000000, 0.000000000000000000, -1.000000000000000000 ) ) ;
#16972=VERTEX_POINT ( 'NONE', #6040 ) ;
#17073=VERTEX_POINT ( 'NONE', #4190 ) ;
#17121=CARTESIAN_POINT ( 'NONE',  ( 89.27853238427192650, -9.950806628697387524, -13.58228004074779705 ) ) ;
#17226=DIRECTION ( 'NONE',  ( -0.8636456077245086016, 0.5040994586965593660, 0.000000000000000000 ) ) ;
#17284=CIRCLE ( 'NONE', #27467, 3.000000000000003997 ) ;
#17306=EDGE_CURVE ( 'NONE', #26554, #14451, #24395, .T. ) ;
#17325=ORIENTED_EDGE ( 'NONE', *, *, #8562, .F. ) ;
#17347=CARTESIAN_POINT ( 'NONE',  ( 82.31000308962319423, -13.76004065658516673, -8.143215200338314474 ) ) ;
#17486=LINE ( 'NONE', #7007, #39493 ) ;
#17554=CARTESIAN_POINT ( 'NONE',  ( 89.19450566478245435, -10.26038732334573744, -13.97729785597371333 ) ) ;
#17562=SURFACE_STYLE_FILL_AREA ( #35081 ) ;
#17596=VERTEX_POINT ( 'NONE', #25743 ) ;
#17665=DIRECTION ( 'NONE',  ( -0.5040994586965557023, -0.8636456077245108220, 0.000000000000000000 ) ) ;
#17696=DIRECTION ( 'NONE',  ( -0.8636456077245086016, 0.5040994586965593660, 0.000000000000000000 ) ) ;
#17709=AXIS2_PLACEMENT_3D ( 'NONE', #39882, #1789, #33244 ) ;
#17728=VECTOR ( 'NONE', #15214, 1000.000000000000000 ) ;
#17777=FACE_OUTER_BOUND ( 'NONE', #39443, .T. ) ;
#17809=CARTESIAN_POINT ( 'NONE',  ( 73.60369002873177635, -5.846784287000932778, -8.143215200338314474 ) ) ;
#17845=ORIENTED_EDGE ( 'NONE', *, *, #16681, .T. ) ;
#17861=ORIENTED_EDGE ( 'NONE', *, *, #42030, .F. ) ;
#17899=ADVANCED_FACE ( 'NONE', ( #26929 ), #2980, .T. ) ;
#18007=CARTESIAN_POINT ( 'NONE',  ( 85.38561350750011059, -9.917550408422661334, -8.143215200338314474 ) ) ;
#18080=AXIS2_PLACEMENT_3D ( 'NONE', #36883, #43978, #5203 ) ;
#18099=ORIENTED_EDGE ( 'NONE', *, *, #16161, .F. ) ;
#18138=CIRCLE ( 'NONE', #20341, 3.000000000000003997 ) ;
#18139=CIRCLE ( 'NONE', #10896, 1.499999999999996225 ) ;
#18186=VERTEX_POINT ( 'NONE', #11436 ) ;
#18224=PLANE ( 'NONE',  #6438 ) ;
#18229=CARTESIAN_POINT ( 'NONE',  ( 88.68444135278477347, -11.19878434816932611, -14.07504941314370406 ) ) ;
#18265=ORIENTED_EDGE ( 'NONE', *, *, #9032, .F. ) ;
#18347=CARTESIAN_POINT ( 'NONE',  ( 88.88468749803642766, -10.91782331763674385, -14.14321520033831625 ) ) ;
#18407=ORIENTED_EDGE ( 'NONE', *, *, #14712, .F. ) ;
#18438=PLANE ( 'NONE',  #22321 ) ;
#18456=DIRECTION ( 'NONE',  ( 0.000000000000000000, 0.000000000000000000, -1.000000000000000000 ) ) ;
#18497=DIRECTION ( 'NONE',  ( 0.8636456077245080465, -0.5040994586965603652, 0.000000000000000000 ) ) ;
#18524=VERTEX_POINT ( 'NONE', #40664 ) ;
#18531=ORIENTED_EDGE ( 'NONE', *, *, #861, .T. ) ;
#18603=ORIENTED_EDGE ( 'NONE', *, *, #3313, .T. ) ;
#18626=EDGE_CURVE ( 'NONE', #6780, #15033, #43236, .T. ) ;
#18631=CIRCLE ( 'NONE', #12083, 1.499999999999996225 ) ;
#18639=CARTESIAN_POINT ( 'NONE',  ( 85.83930302032702286, -9.140269361470597431, -14.14321520033831625 ) ) ;
#18656=( GEOMETRIC_REPRESENTATION_CONTEXT ( 3 ) GLOBAL_UNCERTAINTY_ASSIGNED_CONTEXT ( ( #27891 ) ) GLOBAL_UNIT_ASSIGNED_CONTEXT ( ( #14138, #13313, #27220 ) ) REPRESENTATION_CONTEXT ( 'NONE', 'WORKASPACE' ) );
#18714=CARTESIAN_POINT ( 'NONE',  ( 85.45605303719084134, -15.74807682313488222, -13.39321520033831447 ) ) ;
#18751=VECTOR ( 'NONE', #2389, 1000.000000000000000 ) ;
#18810=LINE ( 'NONE', #28079, #28806 ) ;
#18893=FACE_OUTER_BOUND ( 'NONE', #12105, .T. ) ;
#18898=CARTESIAN_POINT ( 'NONE',  ( 88.69221322696461129, -11.18906686396361749, -14.08003406886638764 ) ) ;
#18906=CYLINDRICAL_SURFACE ( 'NONE', #41656, 3.000000000000003997 ) ;
#18923=EDGE_CURVE ( 'NONE', #36064, #43343, #3911, .T. ) ;
#18966=ORIENTED_EDGE ( 'NONE', *, *, #6669, .T. ) ;
#18978=DIRECTION ( 'NONE',  ( 0.8636456077245090457, -0.5040994586965586999, 0.000000000000000000 ) ) ;
#19021=ORIENTED_EDGE ( 'NONE', *, *, #21715, .F. ) ;
#19108=VERTEX_POINT ( 'NONE', #41018 ) ;
#19118=ORIENTED_EDGE ( 'NONE', *, *, #11080, .T. ) ;
#19146=B_SPLINE_CURVE_WITH_KNOTS ( 'NONE', 3,
 ( #39878, #15035, #28946, #7736, #4307, #36220, #38967, #11169, #18898, #32789, #18229, #42854, #11613, #8643, #22543, #25524, #32573, #35535, #32123, #1340, #15254, #39195, #7961, #42630 ),
 .UNSPECIFIED., .F., .F.,
 ( 4, 2, 2, 1, 1, 2, 2, 2, 2, 2, 2, 2, 4 ),
 ( 0.000000000000000000, 0.1250000000000380806, 0.1875000000000567879, 0.2187500000000661415, 0.2343750000000627276, 0.2421875000000603961, 0.2500000000000580647, 0.3750000000000387468, 0.4375000000000208722, 0.4687500000000185962, 0.5000000000000163203, 0.7500000000000082157, 1.000000000000000000 ),
 .UNSPECIFIED. ) ;
#19178=VECTOR ( 'NONE', #37584, 1000.000000000000000 ) ;
#19233=CARTESIAN_POINT ( 'NONE',  ( 75.95778847736481509, -3.256761025687722189, -18.64321520033831803 ) ) ;
#19235=VERTEX_POINT ( 'NONE', #33516 ) ;
#19264=AXIS2_PLACEMENT_3D ( 'NONE', #36293, #36519, #5292 ) ;
#19475=EDGE_CURVE ( 'NONE', #34692, #14979, #2435, .T. ) ;
#19515=CIRCLE ( 'NONE', #2022, 5.999999999999997335 ) ;
#19566=DIRECTION ( 'NONE',  ( -0.8636456077245086016, 0.5040994586965593660, 0.000000000000000000 ) ) ;
#19586=ORIENTED_EDGE ( 'NONE', *, *, #42601, .T. ) ;
#19646=VECTOR ( 'NONE', #21669, 1000.000000000000000 ) ;
#19650=DIRECTION ( 'NONE',  ( 0.8636456077245092677, -0.5040994586965584778, 0.000000000000000000 ) ) ;
#19817=VERTEX_POINT ( 'NONE', #10947 ) ;
#19821=CARTESIAN_POINT ( 'NONE',  ( 75.95778847736481509, -3.256761025687722189, -7.993215200338315007 ) ) ;
#19850=VERTEX_POINT ( 'NONE', #29393 ) ;
#19855=EDGE_CURVE ( 'NONE', #12781, #9608, #29337, .T. ) ;
#19915=EDGE_LOOP ( 'NONE', ( #41446, #27429, #7142, #24044, #20667, #19021, #40552, #24229, #14004, #31057, #28000 ) ) ;
#20073=EDGE_CURVE ( 'NONE', #36947, #18524, #32252, .T. ) ;
#20090=CARTESIAN_POINT ( 'NONE',  ( 89.28374162313775741, -9.926294987500817513, -13.51696516463038833 ) ) ;
#20132=DIRECTION ( 'NONE',  ( 0.6725995567522981000, 0.7400066460894877407, -0.000000000000000000 ) ) ;
#20205=DIRECTION ( 'NONE',  ( 0.9495615000563050190, -0.3135808629537517600, 0.000000000000000000 ) ) ;
#20232=DIRECTION ( 'NONE',  ( 0.000000000000000000, 0.000000000000000000, 1.000000000000000000 ) ) ;
#20245=CARTESIAN_POINT ( 'NONE',  ( 86.34560043013698305, -9.320000780048239619, -18.64321520033831803 ) ) ;
#20275=EDGE_LOOP ( 'NONE', ( #18099, #24573, #41917, #23693 ) ) ;
#20313=CARTESIAN_POINT ( 'NONE',  ( 89.13434580277143482, -10.42584736732164608, -14.07205986288570010 ) ) ;
#20324=EDGE_LOOP ( 'NONE', ( #26245, #43972 ) ) ;
#20333=EDGE_CURVE ( 'NONE', #34402, #33083, #37803, .T. ) ;
#20341=AXIS2_PLACEMENT_3D ( 'NONE', #7019, #34804, #25473 ) ;
#20347=CARTESIAN_POINT ( 'NONE',  ( 75.95778847736481509, -3.256761025687722189, -8.143215200338314474 ) ) ;
#20400=CARTESIAN_POINT ( 'NONE',  ( 75.95778847736481509, -3.256761025687722189, -8.143215200338314474 ) ) ;
#20407=ORIENTED_EDGE ( 'NONE', *, *, #35055, .F. ) ;
#20410=AXIS2_PLACEMENT_3D ( 'NONE', #44911, #20730, #6139 ) ;
#20447=EDGE_CURVE ( 'NONE', #17073, #34692, #41038, .T. ) ;
#20454=LINE ( 'NONE', #13392, #20810 ) ;
#20457=LINE ( 'NONE', #16353, #6247 ) ;
#20536=CARTESIAN_POINT ( 'NONE',  ( 89.08937694410278141, -10.53878037750923546, -14.12219449423614037 ) ) ;
#20568=DIRECTION ( 'NONE',  ( -0.8636456077245090457, 0.5040994586965585889, 0.000000000000000000 ) ) ;
#20592=CARTESIAN_POINT ( 'NONE',  ( 77.05532149770296257, 0.06670422450934243574, -16.89321520033831447 ) ) ;
#20609=PRODUCT_DEFINITION_FORMATION_WITH_SPECIFIED_SOURCE ( 'ANY', '', #21957, .NOT_KNOWN. ) ;
#20621=ORIENTED_EDGE ( 'NONE', *, *, #19855, .T. ) ;
#20649=FACE_OUTER_BOUND ( 'NONE', #43767, .T. ) ;
#20667=ORIENTED_EDGE ( 'NONE', *, *, #20891, .F. ) ;
#20697=DIRECTION ( 'NONE',  ( 0.7400066460894876297, -0.6725995567522979890, -0.000000000000000000 ) ) ;
#20730=DIRECTION ( 'NONE',  ( 0.000000000000000000, 0.000000000000000000, 1.000000000000000000 ) ) ;
#20758=CARTESIAN_POINT ( 'NONE',  ( 89.13851161028307502, -10.41525819279620357, -14.06723350770984382 ) ) ;
#20773=ORIENTED_EDGE ( 'NONE', *, *, #14051, .T. ) ;
#20810=VECTOR ( 'NONE', #30705, 1000.000000000000000 ) ;
#20891=EDGE_CURVE ( 'NONE', #41111, #36064, #43310, .T. ) ;
#20951=CARTESIAN_POINT ( 'NONE',  ( 90.20794100481921873, -11.57440209418094668, -18.64321520033831803 ) ) ;
#21002=CARTESIAN_POINT ( 'NONE',  ( 77.25325688895158294, -4.012910213732562070, -7.993215200338315007 ) ) ;
#21133=AXIS2_PLACEMENT_3D ( 'NONE', #18714, #8452, #1150 ) ;
#21205=ADVANCED_FACE ( 'NONE', ( #17777 ), #38732, .F. ) ;
#21229=CARTESIAN_POINT ( 'NONE',  ( 85.45605303719084134, -15.74807682313488222, -9.893215200338316251 ) ) ;
#21248=CARTESIAN_POINT ( 'NONE',  ( 86.39381242489322688, -8.190259192973641689, -13.24321520033830879 ) ) ;
#21391=DIRECTION ( 'NONE',  ( 0.000000000000000000, 0.000000000000000000, 1.000000000000000000 ) ) ;
#21425=PRESENTATION_STYLE_ASSIGNMENT (( #31456 ) ) ;
#21430=EDGE_CURVE ( 'NONE', #19108, #17596, #32578, .T. ) ;
#21507=VECTOR ( 'NONE', #5405, 1000.000000000000000 ) ;
#21537=LINE ( 'NONE', #24516, #33443 ) ;
#21574=DIRECTION ( 'NONE',  ( -0.8636456077245086016, 0.5040994586965593660, 0.000000000000000000 ) ) ;
#21578=AXIS2_PLACEMENT_3D ( 'NONE', #12316, #26444, #29632 ) ;
#21595=CARTESIAN_POINT ( 'NONE',  ( 88.22708560785949317, -3.622631779710408395, -9.893215200338316251 ) ) ;
#21649=DIRECTION ( 'NONE',  ( 0.000000000000000000, 0.000000000000000000, 1.000000000000000000 ) ) ;
#21655=ORIENTED_EDGE ( 'NONE', *, *, #21715, .T. ) ;
#21662=ORIENTED_EDGE ( 'NONE', *, *, #15178, .T. ) ;
#21667=ORIENTED_EDGE ( 'NONE', *, *, #23077, .T. ) ;
#21669=DIRECTION ( 'NONE',  ( 0.000000000000000000, 0.000000000000000000, 1.000000000000000000 ) ) ;
#21670=CARTESIAN_POINT ( 'NONE',  ( 77.05532149770296257, 0.06670422450934243574, -18.64321520033831803 ) ) ;
#21676=LINE ( 'NONE', #21229, #36109 ) ;
#21685=EDGE_LOOP ( 'NONE', ( #29023, #21732, #17845, #8634, #14148, #40843 ) ) ;
#21692=VECTOR ( 'NONE', #25895, 1000.000000000000000 ) ;
#21701=CARTESIAN_POINT ( 'NONE',  ( 85.94012291206631460, -8.967540239925705592, -14.14321520033831625 ) ) ;
#21715=EDGE_CURVE ( 'NONE', #14979, #41111, #40800, .T. ) ;
#21732=ORIENTED_EDGE ( 'NONE', *, *, #38095, .T. ) ;
#21881=CIRCLE ( 'NONE', #41564, 5.999999999999997335 ) ;
#21893=VECTOR ( 'NONE', #10439, 1000.000000000000000 ) ;
#21945=EDGE_LOOP ( 'NONE', ( #5302, #20773 ) ) ;
#21957=PRODUCT ( 'Cable Anchor', 'Cable Anchor', '', ( #2639 ) ) ;
#22045=DIRECTION ( 'NONE',  ( 0.8636456077245089347, -0.5040994586965590329, 0.000000000000000000 ) ) ;
#22063=ORIENTED_EDGE ( 'NONE', *, *, #30909, .T. ) ;
#22120=FACE_OUTER_BOUND ( 'NONE', #244, .T. ) ;
#22126=EDGE_CURVE ( 'NONE', #29422, #10447, #848, .T. ) ;
#22152=ORIENTED_EDGE ( 'NONE', *, *, #27340, .F. ) ;
#22166=AXIS2_PLACEMENT_3D ( 'NONE', #10251, #28023, #34171 ) ;
#22184=EDGE_LOOP ( 'NONE', ( #29938, #6493, #22374, #36422 ) ) ;
#22321=AXIS2_PLACEMENT_3D ( 'NONE', #38710, #1093, #28699 ) ;
#22374=ORIENTED_EDGE ( 'NONE', *, *, #32613, .T. ) ;
#22389=DIRECTION ( 'NONE',  ( 0.000000000000000000, 0.000000000000000000, 1.000000000000000000 ) ) ;
#22400=DIRECTION ( 'NONE',  ( 0.000000000000000000, 0.000000000000000000, 1.000000000000000000 ) ) ;
#22414=LINE ( 'NONE', #39293, #43504 ) ;
#22443=ORIENTED_EDGE ( 'NONE', *, *, #2184, .T. ) ;
#22457=ORIENTED_EDGE ( 'NONE', *, *, #21430, .T. ) ;
#22482=DIRECTION ( 'NONE',  ( 0.8636456077245092677, -0.5040994586965584778, 0.000000000000000000 ) ) ;
#22543=CARTESIAN_POINT ( 'NONE',  ( 88.56442385468598388, -11.33890518539517522, -13.97496118938472698 ) ) ;
#22547=LINE ( 'NONE', #8869, #6258 ) ;
#22611=PLANE ( 'NONE',  #42762 ) ;
#22620=EDGE_CURVE ( 'NONE', #34510, #13487, #14109, .T. ) ;
#22660=VERTEX_POINT ( 'NONE', #22954 ) ;
#22759=CARTESIAN_POINT ( 'NONE',  ( 88.22708560785949317, -3.622631779710408395, -18.64321520033831803 ) ) ;
#22776=EDGE_CURVE ( 'NONE', #43318, #34402, #586, .T. ) ;
#22831=CARTESIAN_POINT ( 'NONE',  ( 89.29245855188943892, -9.882163754870950001, -8.143215200338314474 ) ) ;
#22849=VECTOR ( 'NONE', #15788, 1000.000000000000000 ) ;
#22949=CIRCLE ( 'NONE', #33838, 5.999999999999997335 ) ;
#22954=CARTESIAN_POINT ( 'NONE',  ( 77.25325688895158294, -4.012910213732562070, -8.143215200338314474 ) ) ;
#22960=( NAMED_UNIT ( * ) SI_UNIT ( $, .STERADIAN. ) SOLID_ANGLE_UNIT ( ) );
#22984=CYLINDRICAL_SURFACE ( 'NONE', #9358, 5.999999999999997335 ) ;
#23077=EDGE_CURVE ( 'NONE', #10999, #41325, #7566, .T. ) ;
#23129=EDGE_LOOP ( 'NONE', ( #15383, #21667 ) ) ;
#23190=ORIENTED_EDGE ( 'NONE', *, *, #14712, .T. ) ;
#23253=LINE ( 'NONE', #15505, #14643 ) ;
#23302=APPLICATION_CONTEXT ( 'automotive_design' ) ;
#23483=CARTESIAN_POINT ( 'NONE',  ( 75.95778847736481509, -3.256761025687722189, -9.893215200338316251 ) ) ;
#23490=CARTESIAN_POINT ( 'NONE',  ( 82.31000308962319423, -13.76004065658516673, -18.64321520033831803 ) ) ;
#23502=CIRCLE ( 'NONE', #31481, 1.499999999999996225 ) ;
#23615=LINE ( 'NONE', #33612, #18751 ) ;
#23693=ORIENTED_EDGE ( 'NONE', *, *, #31684, .T. ) ;
#23771=CARTESIAN_POINT ( 'NONE',  ( 85.38561350750011059, -9.917550408422661334, -13.24321520033830879 ) ) ;
#23783=DIRECTION ( 'NONE',  ( -0.9495615000563050190, 0.3135808629537517600, 0.000000000000000000 ) ) ;
#23822=ADVANCED_FACE ( 'NONE', ( #32537, #25935 ), #32086, .F. ) ;
#23853=DIRECTION ( 'NONE',  ( 0.8636456077245089347, -0.5040994586965590329, 0.000000000000000000 ) ) ;
#23890=CARTESIAN_POINT ( 'NONE',  ( 88.28425963449632263, -11.60945497031996787, -18.64321520033831803 ) ) ;
#23908=ORIENTED_EDGE ( 'NONE', *, *, #18626, .F. ) ;
#23964=CARTESIAN_POINT ( 'NONE',  ( 89.23646529747401246, -10.12233672812908480, -13.85167412278761923 ) ) ;
#24039=ORIENTED_EDGE ( 'NONE', *, *, #37414, .T. ) ;
#24044=ORIENTED_EDGE ( 'NONE', *, *, #9731, .F. ) ;
#24063=ORIENTED_EDGE ( 'NONE', *, *, #9731, .T. ) ;
#24229=ORIENTED_EDGE ( 'NONE', *, *, #31988, .F. ) ;
#24242=VECTOR ( 'NONE', #10715, 1000.000000000000000 ) ;
#24313=ADVANCED_FACE ( 'NONE', ( #34554 ), #24322, .F. ) ;
#24322=PLANE ( 'NONE',  #34226 ) ;
#24395=LINE ( 'NONE', #37453, #24242 ) ;
#24516=CARTESIAN_POINT ( 'NONE',  ( 91.23658249893594530, -5.844616714554617509, -18.64321520033831803 ) ) ;
#24573=ORIENTED_EDGE ( 'NONE', *, *, #21430, .F. ) ;
#24580=CIRCLE ( 'NONE', #36215, 0.8999999999999980238 ) ;
#24620=CARTESIAN_POINT ( 'NONE',  ( 89.25811708600326710, -10.04048109355869300, -13.74760083314252768 ) ) ;
#24743=EDGE_CURVE ( 'NONE', #32138, #44381, #27412, .T. ) ;
#24796=CIRCLE ( 'NONE', #14605, 3.500000000000003109 ) ;
#24813=CARTESIAN_POINT ( 'NONE',  ( 75.95778847736481509, -3.256761025687722189, -16.89321520033831447 ) ) ;
#24861=EDGE_CURVE ( 'NONE', #38458, #10189, #24796, .T. ) ;
#24935=AXIS2_PLACEMENT_3D ( 'NONE', #36666, #30293, #11847 ) ;
#24964=EDGE_LOOP ( 'NONE', ( #11382, #37937, #22152, #2562, #33600, #8380, #44387, #36729 ) ) ;
#25080=PLANE ( 'NONE',  #38299 ) ;
#25083=ORIENTED_EDGE ( 'NONE', *, *, #9602, .T. ) ;
#25093=AXIS2_PLACEMENT_3D ( 'NONE', #37033, #5802, #12900 ) ;
#25144=CYLINDRICAL_SURFACE ( 'NONE', #1843, 1.499999999999996225 ) ;
#25230=CIRCLE ( 'NONE', #4088, 3.500000000000003109 ) ;
#25251=CIRCLE ( 'NONE', #5565, 1.499999999999996225 ) ;
#25311=EDGE_LOOP ( 'NONE', ( #22457, #3489, #28363, #41371 ) ) ;
#25319=EDGE_CURVE ( 'NONE', #38775, #19108, #23253, .T. ) ;
#25399=ORIENTED_EDGE ( 'NONE', *, *, #15908, .F. ) ;
#25451=ORIENTED_EDGE ( 'NONE', *, *, #44531, .F. ) ;
#25473=DIRECTION ( 'NONE',  ( -0.8636456077245092677, 0.5040994586965584778, 0.000000000000000000 ) ) ;
#25524=CARTESIAN_POINT ( 'NONE',  ( 88.53603805838689311, -11.36969738595376000, -13.94316338922722665 ) ) ;
#25529=FACE_OUTER_BOUND ( 'NONE', #31231, .T. ) ;
#25530=CARTESIAN_POINT ( 'NONE',  ( 86.34560043013698305, -9.320000780048239619, -18.64321520033831803 ) ) ;
#25571=ADVANCED_FACE ( 'NONE', ( #43552 ), #12320, .T. ) ;
#25596=EDGE_CURVE ( 'NONE', #14979, #36847, #9119, .T. ) ;
#25652=CARTESIAN_POINT ( 'NONE',  ( 75.95778847736481509, -3.256761025687722189, -7.993215200338315007 ) ) ;
#25693=EDGE_CURVE ( 'NONE', #38837, #36947, #33283, .T. ) ;
#25717=LINE ( 'NONE', #39847, #21507 ) ;
#25738=EDGE_CURVE ( 'NONE', #19235, #37757, #37788, .T. ) ;
#25743=CARTESIAN_POINT ( 'NONE',  ( 73.60369002873177635, -5.846784287000932778, -16.89321520033831447 ) ) ;
#25845=CIRCLE ( 'NONE', #10567, 5.999999999999997335 ) ;
#25888=DIRECTION ( 'NONE',  ( 0.000000000000000000, 0.000000000000000000, -1.000000000000000000 ) ) ;
#25895=DIRECTION ( 'NONE',  ( 0.000000000000000000, 0.000000000000000000, -1.000000000000000000 ) ) ;
#25929=AXIS2_PLACEMENT_3D ( 'NONE', #12402, #15590, #26302 ) ;
#25931=ORIENTED_EDGE ( 'NONE', *, *, #27571, .T. ) ;
#25935=FACE_OUTER_BOUND ( 'NONE', #34410, .T. ) ;
#25958=CYLINDRICAL_SURFACE ( 'NONE', #43039, 3.500000000000003109 ) ;
#25989=DIRECTION ( 'NONE',  ( -0.8636456077245092677, 0.5040994586965584778, 0.000000000000000000 ) ) ;
#26006=CARTESIAN_POINT ( 'NONE',  ( 86.34560043013698305, -9.320000780048239619, -9.893215200338316251 ) ) ;
#26066=ORIENTED_EDGE ( 'NONE', *, *, #24861, .T. ) ;
#26105=ORIENTED_EDGE ( 'NONE', *, *, #27633, .T. ) ;
#26109=CARTESIAN_POINT ( 'NONE',  ( 77.25325688895158294, -4.012910213732562070, -18.64321520033831803 ) ) ;
#26219=DIRECTION ( 'NONE',  ( 0.000000000000000000, 0.000000000000000000, -1.000000000000000000 ) ) ;
#26240=DIRECTION ( 'NONE',  ( 0.8636456077245090457, -0.5040994586965586999, 0.000000000000000000 ) ) ;
#26245=ORIENTED_EDGE ( 'NONE', *, *, #42975, .F. ) ;
#26250=SHAPE_REPRESENTATION ( 'Cable Anchor', ( #12375 ), #18656 ) ;
#26302=DIRECTION ( 'NONE',  ( -0.8636456077245080465, 0.5040994586965603652, 0.000000000000000000 ) ) ;
#26334=CARTESIAN_POINT ( 'NONE',  ( 75.95778847736481509, -3.256761025687722189, -9.893215200338316251 ) ) ;
#26420=EDGE_CURVE ( 'NONE', #29422, #32138, #19146, .T. ) ;
#26444=DIRECTION ( 'NONE',  ( 0.8636456077245089347, -0.5040994586965589219, 0.000000000000000000 ) ) ;
#26554=VERTEX_POINT ( 'NONE', #34088 ) ;
#26592=ORIENTED_EDGE ( 'NONE', *, *, #20333, .T. ) ;
#26726=FACE_OUTER_BOUND ( 'NONE', #9331, .T. ) ;
#26766=DIRECTION ( 'NONE',  ( 0.000000000000000000, 0.000000000000000000, 1.000000000000000000 ) ) ;
#26792=CARTESIAN_POINT ( 'NONE',  ( 86.34560043013698305, -9.320000780048239619, -16.89321520033831447 ) ) ;
#26887=EDGE_LOOP ( 'NONE', ( #12736, #742, #44842, #29349 ) ) ;
#26929=FACE_OUTER_BOUND ( 'NONE', #22184, .T. ) ;
#26961=DIRECTION ( 'NONE',  ( 0.000000000000000000, 0.000000000000000000, 1.000000000000000000 ) ) ;
#26982=CARTESIAN_POINT ( 'NONE',  ( 90.15753105894957287, -11.66076665495339348, -14.14321520033831625 ) ) ;
#27036=DIRECTION ( 'NONE',  ( -0.8636456077245080465, 0.5040994586965603652, 0.000000000000000000 ) ) ;
#27152=CARTESIAN_POINT ( 'NONE',  ( 89.29151511389673601, -9.887673028482419468, -13.35680558263691609 ) ) ;
#27213=VECTOR ( 'NONE', #43538, 1000.000000000000000 ) ;
#27220=( NAMED_UNIT ( * ) SI_UNIT ( $, .STERADIAN. ) SOLID_ANGLE_UNIT ( ) );
#27340=EDGE_CURVE ( 'NONE', #16620, #18524, #42875, .T. ) ;
#27404=ORIENTED_EDGE ( 'NONE', *, *, #32901, .F. ) ;
#27412=LINE ( 'NONE', #23771, #2195 ) ;
#27429=ORIENTED_EDGE ( 'NONE', *, *, #30362, .T. ) ;
#27443=AXIS2_PLACEMENT_3D ( 'NONE', #1835, #8920, #5937 ) ;
#27467=AXIS2_PLACEMENT_3D ( 'NONE', #83, #32206, #4169 ) ;
#27567=EDGE_LOOP ( 'NONE', ( #25399, #30041, #37244, #29909 ) ) ;
#27571=EDGE_CURVE ( 'NONE', #43318, #26554, #38259, .T. ) ;
#27599=ORIENTED_EDGE ( 'NONE', *, *, #18923, .F. ) ;
#27605=CARTESIAN_POINT ( 'NONE',  ( 89.16143781654311340, -10.35449676759526305, -14.03636009902034409 ) ) ;
#27617=CARTESIAN_POINT ( 'NONE',  ( 74.66232006577804725, -2.500611837642884527, -18.64321520033831803 ) ) ;
#27633=EDGE_CURVE ( 'NONE', #5895, #37436, #2921, .T. ) ;
#27673=VERTEX_POINT ( 'NONE', #20592 ) ;
#27715=CARTESIAN_POINT ( 'NONE',  ( 88.19154317003298615, -15.02898452507898241, -8.143215200338314474 ) ) ;
#27891=UNCERTAINTY_MEASURE_WITH_UNIT (LENGTH_MEASURE( 1.000000000000000082E-05 ), #14138, 'distance_accuracy_value', 'NONE');
#27952=AXIS2_PLACEMENT_3D ( 'NONE', #30571, #9838, #44948 ) ;
#27975=DIRECTION ( 'NONE',  ( 0.8636456077245088236, -0.5040994586965589219, 0.000000000000000000 ) ) ;
#28000=ORIENTED_EDGE ( 'NONE', *, *, #28388, .T. ) ;
#28023=DIRECTION ( 'NONE',  ( 0.000000000000000000, 0.000000000000000000, -1.000000000000000000 ) ) ;
#28047=CARTESIAN_POINT ( 'NONE',  ( 88.98550738977573360, -10.74509419609185379, -14.14321520033831625 ) ) ;
#28078=DIRECTION ( 'NONE',  ( 0.8636456077245088236, -0.5040994586965589219, 0.000000000000000000 ) ) ;
#28079=CARTESIAN_POINT ( 'NONE',  ( 88.22708560785949317, -3.622631779710408395, -18.64321520033831803 ) ) ;
#28088=CIRCLE ( 'NONE', #8426, 3.500000000000003109 ) ;
#28225=LINE ( 'NONE', #32070, #40742 ) ;
#28323=ORIENTED_EDGE ( 'NONE', *, *, #42975, .T. ) ;
#28363=ORIENTED_EDGE ( 'NONE', *, *, #36724, .F. ) ;
#28388=EDGE_CURVE ( 'NONE', #37757, #41378, #41542, .T. ) ;
#28397=AXIS2_PLACEMENT_3D ( 'NONE', #26006, #29419, #15742 ) ;
#28422=CARTESIAN_POINT ( 'NONE',  ( 86.34560043013698305, -9.320000780048239619, -8.143215200338314474 ) ) ;
#28502=CARTESIAN_POINT ( 'NONE',  ( 75.95778847736481509, -3.256761025687722189, -7.993215200338315007 ) ) ;
#28503=( NAMED_UNIT ( * ) SI_UNIT ( $, .STERADIAN. ) SOLID_ANGLE_UNIT ( ) );
#28506=DIRECTION ( 'NONE',  ( -0.8636456077245089347, 0.5040994586965589219, 0.000000000000000000 ) ) ;
#28509=ORIENTED_EDGE ( 'NONE', *, *, #34790, .T. ) ;
#28565=DIRECTION ( 'NONE',  ( -0.8636456077245080465, 0.5040994586965603652, 0.000000000000000000 ) ) ;
#28571=LINE ( 'NONE', #11242, #9886 ) ;
#28622=ORIENTED_EDGE ( 'NONE', *, *, #38409, .T. ) ;
#28693=DIRECTION ( 'NONE',  ( 0.8636456077245090457, -0.5040994586965586999, 0.000000000000000000 ) ) ;
#28699=DIRECTION ( 'NONE',  ( 0.000000000000000000, 0.000000000000000000, -1.000000000000000000 ) ) ;
#28713=ORIENTED_EDGE ( 'NONE', *, *, #16105, .T. ) ;
#28743=ORIENTED_EDGE ( 'NONE', *, *, #40151, .T. ) ;
#28746=DIRECTION ( 'NONE',  ( 0.000000000000000000, 0.000000000000000000, 1.000000000000000000 ) ) ;
#28759=EDGE_CURVE ( 'NONE', #10189, #38611, #44151, .T. ) ;
#28806=VECTOR ( 'NONE', #31260, 1000.000000000000114 ) ;
#28828=ORIENTED_EDGE ( 'NONE', *, *, #32901, .T. ) ;
#28927=CARTESIAN_POINT ( 'NONE',  ( 83.75466360696344736, -7.807702403958562520, -18.64321520033831803 ) ) ;
#28946=CARTESIAN_POINT ( 'NONE',  ( 88.82299970795220645, -11.01275678708395489, -14.13803923971916632 ) ) ;
#28956=DIRECTION ( 'NONE',  ( 0.8636456077245092677, -0.5040994586965584778, 0.000000000000000000 ) ) ;
#29023=ORIENTED_EDGE ( 'NONE', *, *, #10840, .T. ) ;
#29126=DIRECTION ( 'NONE',  ( 0.5040994586965589219, 0.8636456077245089347, 0.000000000000000000 ) ) ;
#29128=CARTESIAN_POINT ( 'NONE',  ( 75.95778847736481509, -3.256761025687722189, -7.993215200338315007 ) ) ;
#29162=DIRECTION ( 'NONE',  ( 0.000000000000000000, 0.000000000000000000, -1.000000000000000000 ) ) ;
#29246=LINE ( 'NONE', #39953, #16481 ) ;
#29297=AXIS2_PLACEMENT_3D ( 'NONE', #7781, #7547, #18497 ) ;
#29337=CIRCLE ( 'NONE', #24935, 5.999999999999997335 ) ;
#29349=ORIENTED_EDGE ( 'NONE', *, *, #14051, .F. ) ;
#29393=CARTESIAN_POINT ( 'NONE',  ( 88.22708560785949317, -3.622631779710408395, -16.89321520033831447 ) ) ;
#29419=DIRECTION ( 'NONE',  ( 0.000000000000000000, 0.000000000000000000, 1.000000000000000000 ) ) ;
#29422=VERTEX_POINT ( 'NONE', #18347 ) ;
#29458=EDGE_LOOP ( 'NONE', ( #24063, #18531, #13214, #28509, #27599 ) ) ;
#29538=EDGE_LOOP ( 'NONE', ( #38820, #41090, #3438, #26105 ) ) ;
#29548=CARTESIAN_POINT ( 'NONE',  ( 73.60369002873177635, -5.846784287000932778, -18.64321520033831803 ) ) ;
#29632=DIRECTION ( 'NONE',  ( 0.000000000000000000, 0.000000000000000000, 1.000000000000000000 ) ) ;
#29658=CYLINDRICAL_SURFACE ( 'NONE', #8836, 3.500000000000003109 ) ;
#29752=FACE_OUTER_BOUND ( 'NONE', #6369, .T. ) ;
#29769=CARTESIAN_POINT ( 'NONE',  ( 75.95778847736481509, -3.256761025687722189, -7.993215200338315007 ) ) ;
#29770=CARTESIAN_POINT ( 'NONE',  ( 82.31000308962319423, -13.76004065658516673, -18.64321520033831803 ) ) ;
#29804=FACE_OUTER_BOUND ( 'NONE', #29538, .T. ) ;
#29827=CARTESIAN_POINT ( 'NONE',  ( 86.34560043013698305, -9.320000780048239619, -18.64321520033831803 ) ) ;
#29837=EDGE_CURVE ( 'NONE', #44995, #38458, #224, .T. ) ;
#29838=EDGE_LOOP ( 'NONE', ( #42896, #19118, #30703, #3683, #33879, #16900, #39035, #43819, #1711 ) ) ;
#29851=ORIENTED_EDGE ( 'NONE', *, *, #2037, .T. ) ;
#29852=ADVANCED_FACE ( 'NONE', ( #34422 ), #6630, .T. ) ;
#29862=CARTESIAN_POINT ( 'NONE',  ( 90.71204046351577688, -10.71075648645643774, -8.143215200338314474 ) ) ;
#29909=ORIENTED_EDGE ( 'NONE', *, *, #36724, .T. ) ;
#29938=ORIENTED_EDGE ( 'NONE', *, *, #3313, .F. ) ;
#29998=PLANE ( 'NONE',  #7766 ) ;
#30041=ORIENTED_EDGE ( 'NONE', *, *, #45087, .F. ) ;
#30115=ADVANCED_FACE ( 'NONE', ( #7738 ), #446, .T. ) ;
#30293=DIRECTION ( 'NONE',  ( 0.000000000000000000, 0.000000000000000000, 1.000000000000000000 ) ) ;
#30304=CARTESIAN_POINT ( 'NONE',  ( 87.62389663665700823, -12.03403077406018440, -9.893215200338316251 ) ) ;
#30362=EDGE_CURVE ( 'NONE', #44507, #34894, #2984, .T. ) ;
#30448=DIRECTION ( 'NONE',  ( 0.000000000000000000, 0.000000000000000000, -1.000000000000000000 ) ) ;
#30510=ORIENTED_EDGE ( 'NONE', *, *, #22620, .T. ) ;
#30528=FACE_OUTER_BOUND ( 'NONE', #20324, .T. ) ;
#30556=CARTESIAN_POINT ( 'NONE',  ( 88.93653725331050452, -10.83229915613791761, -18.64321520033831803 ) ) ;
#30571=CARTESIAN_POINT ( 'NONE',  ( 86.34560043013698305, -9.320000780048239619, -8.143215200338314474 ) ) ;
#30703=ORIENTED_EDGE ( 'NONE', *, *, #36407, .T. ) ;
#30705=DIRECTION ( 'NONE',  ( 0.000000000000000000, 0.000000000000000000, 1.000000000000000000 ) ) ;
#30909=EDGE_CURVE ( 'NONE', #41111, #14177, #7329, .T. ) ;
#31010=CARTESIAN_POINT ( 'NONE',  ( 89.26958058349273983, -9.992926966327468463, -13.67320616139556400 ) ) ;
#31022=CARTESIAN_POINT ( 'NONE',  ( 87.62389663665700823, -12.03403077406018440, -16.89321520033831447 ) ) ;
#31057=ORIENTED_EDGE ( 'NONE', *, *, #25738, .T. ) ;
#31142=AXIS2_PLACEMENT_3D ( 'NONE', #15402, #25888, #8336 ) ;
#31153=DIRECTION ( 'NONE',  ( 0.8636456077245088236, -0.5040994586965589219, 0.000000000000000000 ) ) ;
#31156=ADVANCED_FACE ( 'NONE', ( #36489 ), #29658, .T. ) ;
#31231=EDGE_LOOP ( 'NONE', ( #31848, #32517, #9458, #7209 ) ) ;
#31260=DIRECTION ( 'NONE',  ( 0.9495615000563050190, -0.3135808629537517600, 0.000000000000000000 ) ) ;
#31448=CARTESIAN_POINT ( 'NONE',  ( 89.14456494507275863, -10.39963736880928380, -14.05985968316478640 ) ) ;
#31456=SURFACE_STYLE_USAGE ( .BOTH. , #35540 ) ;
#31463=LINE ( 'NONE', #34211, #38722 ) ;
#31481=AXIS2_PLACEMENT_3D ( 'NONE', #8434, #39670, #7979 ) ;
#31491=LINE ( 'NONE', #34888, #12546 ) ;
#31551=ORIENTED_EDGE ( 'NONE', *, *, #16681, .F. ) ;
#31684=EDGE_CURVE ( 'NONE', #38775, #16972, #882, .T. ) ;
#31725=DIRECTION ( 'NONE',  ( 0.8636456077245088236, -0.5040994586965589219, 0.000000000000000000 ) ) ;
#31747=FACE_OUTER_BOUND ( 'NONE', #8941, .T. ) ;
#31749=EDGE_LOOP ( 'NONE', ( #37764, #5826, #42693, #44964 ) ) ;
#31848=ORIENTED_EDGE ( 'NONE', *, *, #39322, .T. ) ;
#31988=EDGE_CURVE ( 'NONE', #8204, #34692, #11821, .T. ) ;
#32070=CARTESIAN_POINT ( 'NONE',  ( 88.22708560785949317, -3.622631779710408395, -9.893215200338316251 ) ) ;
#32085=ORIENTED_EDGE ( 'NONE', *, *, #20447, .F. ) ;
#32086=PLANE ( 'NONE',  #40793 ) ;
#32123=CARTESIAN_POINT ( 'NONE',  ( 88.49587816393574258, -11.41200697344714143, -13.89319073456437792 ) ) ;
#32135=VECTOR ( 'NONE', #14860, 1000.000000000000000 ) ;
#32138=VERTEX_POINT ( 'NONE', #7484 ) ;
#32206=DIRECTION ( 'NONE',  ( 0.000000000000000000, 0.000000000000000000, 1.000000000000000000 ) ) ;
#32252=CIRCLE ( 'NONE', #17709, 5.999999999999997335 ) ;
#32280=EDGE_CURVE ( 'NONE', #523, #9906, #23502, .T. ) ;
#32283=EDGE_CURVE ( 'NONE', #34894, #44507, #11840, .T. ) ;
#32446=DIRECTION ( 'NONE',  ( -0.8636456077245080465, 0.5040994586965603652, 0.000000000000000000 ) ) ;
#32474=AXIS2_PLACEMENT_3D ( 'NONE', #25530, #38513, #35995 ) ;
#32517=ORIENTED_EDGE ( 'NONE', *, *, #37552, .F. ) ;
#32518=CARTESIAN_POINT ( 'NONE',  ( 74.66232006577804725, -2.500611837642884527, -7.993215200338315007 ) ) ;
#32537=FACE_BOUND ( 'NONE', #21945, .T. ) ;
#32573=CARTESIAN_POINT ( 'NONE',  ( 88.52634549546732501, -11.38007610471903419, -13.93176785127966966 ) ) ;
#32578=LINE ( 'NONE', #39204, #260 ) ;
#32588=ADVANCED_FACE ( 'NONE', ( #30528 ), #36457, .F. ) ;
#32613=EDGE_CURVE ( 'NONE', #15033, #13487, #2479, .T. ) ;
#32627=ORIENTED_EDGE ( 'NONE', *, *, #27633, .F. ) ;
#32644=VERTEX_POINT ( 'NONE', #30304 ) ;
#32755=DIRECTION ( 'NONE',  ( -0.8636456077245080465, 0.5040994586965603652, 0.000000000000000000 ) ) ;
#32789=CARTESIAN_POINT ( 'NONE',  ( 88.68764736394132342, -11.19478773543180239, -14.07713050782770026 ) ) ;
#32811=VECTOR ( 'NONE', #9138, 1000.000000000000114 ) ;
#32901=EDGE_CURVE ( 'NONE', #36847, #14451, #12482, .T. ) ;
#32936=EDGE_LOOP ( 'NONE', ( #21655, #22063, #41967, #4067 ) ) ;
#33071=CIRCLE ( 'NONE', #12731, 3.000000000000003997 ) ;
#33083=VERTEX_POINT ( 'NONE', #9968 ) ;
#33116=DIRECTION ( 'NONE',  ( 0.000000000000000000, 0.000000000000000000, -1.000000000000000000 ) ) ;
#33195=VECTOR ( 'NONE', #38134, 1000.000000000000000 ) ;
#33196=DIRECTION ( 'NONE',  ( -0.8636456077245080465, 0.5040994586965603652, 0.000000000000000000 ) ) ;
#33211=AXIS2_PLACEMENT_3D ( 'NONE', #15559, #36295, #4842 ) ;
#33244=DIRECTION ( 'NONE',  ( 0.8636456077245086016, -0.5040994586965593660, 0.000000000000000000 ) ) ;
#33283=LINE ( 'NONE', #36929, #32811 ) ;
#33390=CARTESIAN_POINT ( 'NONE',  ( 74.66232006577804725, -2.500611837642884527, -9.893215200338316251 ) ) ;
#33443=VECTOR ( 'NONE', #14698, 1000.000000000000000 ) ;
#33516=CARTESIAN_POINT ( 'NONE',  ( 89.33740294208338639, -9.098375579515472822, -9.893215200338316251 ) ) ;
#33585=EDGE_LOOP ( 'NONE', ( #43353, #30510 ) ) ;
#33600=ORIENTED_EDGE ( 'NONE', *, *, #31684, .F. ) ;
#33612=CARTESIAN_POINT ( 'NONE',  ( 89.70384154612264638, -12.43804770190545561, -8.143215200338314474 ) ) ;
#33692=ORIENTED_EDGE ( 'NONE', *, *, #20891, .T. ) ;
#33768=VERTEX_POINT ( 'NONE', #36341 ) ;
#33838=AXIS2_PLACEMENT_3D ( 'NONE', #39570, #4455, #17696 ) ;
#33879=ORIENTED_EDGE ( 'NONE', *, *, #20073, .F. ) ;
#33951=CARTESIAN_POINT ( 'NONE',  ( 73.60369002873177635, -5.846784287000932778, -9.893215200338316251 ) ) ;
#33963=VECTOR ( 'NONE', #6547, 1000.000000000000000 ) ;
#33976=CARTESIAN_POINT ( 'NONE',  ( 89.28011985346235235, -9.943418426816830191, -13.56419841707012708 ) ) ;
#33977=ORIENTED_EDGE ( 'NONE', *, *, #42030, .T. ) ;
#33989=CIRCLE ( 'NONE', #27443, 5.999999999999997335 ) ;
#34018=PLANE ( 'NONE',  #34372 ) ;
#34041=( NAMED_UNIT ( * ) PLANE_ANGLE_UNIT ( ) SI_UNIT ( $, .RADIAN. ) );
#34088=CARTESIAN_POINT ( 'NONE',  ( 92.22433883960545131, -8.119819663282910938, -18.64321520033831803 ) ) ;
#34112=ADVANCED_BREP_SHAPE_REPRESENTATION ( '', ( #6132, #12375 ), #18656 ) ;
#34171=DIRECTION ( 'NONE',  ( -0.8636456077245092677, 0.5040994586965584778, 0.000000000000000000 ) ) ;
#34211=CARTESIAN_POINT ( 'NONE',  ( 85.45605303719084134, -15.74807682313488222, -16.89321520033831447 ) ) ;
#34222=ORIENTED_EDGE ( 'NONE', *, *, #39322, .F. ) ;
#34226=AXIS2_PLACEMENT_3D ( 'NONE', #38640, #41655, #10414 ) ;
#34270=ADVANCED_FACE ( 'NONE', ( #35929 ), #29998, .F. ) ;
#34275=CARTESIAN_POINT ( 'NONE',  ( 75.95778847736481509, -3.256761025687722189, -9.893215200338316251 ) ) ;
#34372=AXIS2_PLACEMENT_3D ( 'NONE', #44077, #20132, #26961 ) ;
#34386=ORIENTED_EDGE ( 'NONE', *, *, #18923, .T. ) ;
#34402=VERTEX_POINT ( 'NONE', #27715 ) ;
#34410=EDGE_LOOP ( 'NONE', ( #26592, #8095, #16794, #38193, #39275, #28828, #14850, #34463, #11689, #41313, #42873 ) ) ;
#34416=CARTESIAN_POINT ( 'NONE',  ( 89.24253794056055256, -10.10023911675148334, -13.82618190763190036 ) ) ;
#34422=FACE_OUTER_BOUND ( 'NONE', #9590, .T. ) ;
#34429=DIRECTION ( 'NONE',  ( 0.5040994586965589219, 0.8636456077245088236, 0.000000000000000000 ) ) ;
#34463=ORIENTED_EDGE ( 'NONE', *, *, #28759, .F. ) ;
#34510=VERTEX_POINT ( 'NONE', #3083 ) ;
#34554=FACE_OUTER_BOUND ( 'NONE', #27567, .T. ) ;
#34649=DIRECTION ( 'NONE',  ( 0.000000000000000000, 0.000000000000000000, 1.000000000000000000 ) ) ;
#34692=VERTEX_POINT ( 'NONE', #1447 ) ;
#34790=EDGE_CURVE ( 'NONE', #10447, #43343, #12635, .T. ) ;
#34804=DIRECTION ( 'NONE',  ( 0.000000000000000000, 0.000000000000000000, -1.000000000000000000 ) ) ;
#34888=CARTESIAN_POINT ( 'NONE',  ( 88.22708560785949317, -3.622631779710408395, -16.89321520033831447 ) ) ;
#34894=VERTEX_POINT ( 'NONE', #30556 ) ;
#35020=DIRECTION ( 'NONE',  ( -0.9495615000563050190, 0.3135808629537517600, 0.000000000000000000 ) ) ;
#35055=EDGE_CURVE ( 'NONE', #14177, #36847, #16354, .T. ) ;
#35081=FILL_AREA_STYLE ('',( #14585 ) ) ;
#35262=ORIENTED_EDGE ( 'NONE', *, *, #4120, .F. ) ;
#35449=DIRECTION ( 'NONE',  ( 0.000000000000000000, 0.000000000000000000, 1.000000000000000000 ) ) ;
#35495=ORIENTED_EDGE ( 'NONE', *, *, #24743, .T. ) ;
#35505=CARTESIAN_POINT ( 'NONE',  ( 88.93653725331050452, -10.83229915613791761, -14.14321520033831625 ) ) ;
#35517=ORIENTED_EDGE ( 'NONE', *, *, #36407, .F. ) ;
#35535=CARTESIAN_POINT ( 'NONE',  ( 88.50659967646818416, -11.40089054768302468, -13.90724332495447868 ) ) ;
#35540=SURFACE_SIDE_STYLE ('',( #17562 ) ) ;
#35572=ORIENTED_EDGE ( 'NONE', *, *, #861, .F. ) ;
#35679=DIRECTION ( 'NONE',  ( 0.000000000000000000, 0.000000000000000000, 1.000000000000000000 ) ) ;
#35762=DIRECTION ( 'NONE',  ( 0.000000000000000000, 0.000000000000000000, -1.000000000000000000 ) ) ;
#35895=EDGE_CURVE ( 'NONE', #44381, #10447, #3950, .T. ) ;
#35929=FACE_OUTER_BOUND ( 'NONE', #31749, .T. ) ;
#35938=DIRECTION ( 'NONE',  ( -0.5040994586965557023, -0.8636456077245108220, 0.000000000000000000 ) ) ;
#35976=DIRECTION ( 'NONE',  ( 0.8636456077245090457, -0.5040994586965586999, 0.000000000000000000 ) ) ;
#35995=DIRECTION ( 'NONE',  ( 0.8636456077245092677, -0.5040994586965584778, 0.000000000000000000 ) ) ;
#36006=CARTESIAN_POINT ( 'NONE',  ( 86.34560043013698305, -9.320000780048239619, -18.64321520033831803 ) ) ;
#36064=VERTEX_POINT ( 'NONE', #4838 ) ;
#36109=VECTOR ( 'NONE', #39225, 1000.000000000000000 ) ;
#36138=ORIENTED_EDGE ( 'NONE', *, *, #27340, .T. ) ;
#36150=DIRECTION ( 'NONE',  ( 0.000000000000000000, 0.000000000000000000, 1.000000000000000000 ) ) ;
#36215=AXIS2_PLACEMENT_3D ( 'NONE', #14058, #27975, #41880 ) ;
#36220=CARTESIAN_POINT ( 'NONE',  ( 88.72832861070837396, -11.14280042575103558, -14.10090787152131320 ) ) ;
#36251=ADVANCED_FACE ( 'NONE', ( #8715, #26726 ), #1857, .T. ) ;
#36284=CARTESIAN_POINT ( 'NONE',  ( 83.32100367795761997, -14.50187442639529323, -9.893215200338316251 ) ) ;
#36293=CARTESIAN_POINT ( 'NONE',  ( 83.32100367795761997, -14.50187442639529323, -16.89321520033831447 ) ) ;
#36295=DIRECTION ( 'NONE',  ( 0.000000000000000000, 0.000000000000000000, -1.000000000000000000 ) ) ;
#36341=CARTESIAN_POINT ( 'NONE',  ( 77.05532149770296257, 0.06670422450934243574, -18.64321520033831803 ) ) ;
#36377=CARTESIAN_POINT ( 'NONE',  ( 87.62389663665700823, -12.03403077406018440, -18.64321520033831803 ) ) ;
#36407=EDGE_CURVE ( 'NONE', #8204, #32644, #33071, .T. ) ;
#36422=ORIENTED_EDGE ( 'NONE', *, *, #22620, .F. ) ;
#36457=PLANE ( 'NONE',  #43875 ) ;
#36489=FACE_OUTER_BOUND ( 'NONE', #25311, .T. ) ;
#36519=DIRECTION ( 'NONE',  ( 0.000000000000000000, 0.000000000000000000, 1.000000000000000000 ) ) ;
#36624=CARTESIAN_POINT ( 'NONE',  ( 90.20794100481921873, -11.57440209418094668, -8.143215200338314474 ) ) ;
#36628=DIRECTION ( 'NONE',  ( 0.000000000000000000, 0.000000000000000000, -1.000000000000000000 ) ) ;
#36666=CARTESIAN_POINT ( 'NONE',  ( 86.34560043013698305, -9.320000780048239619, -9.893215200338316251 ) ) ;
#36676=DIRECTION ( 'NONE',  ( 0.000000000000000000, 0.000000000000000000, -1.000000000000000000 ) ) ;
#36724=EDGE_CURVE ( 'NONE', #33768, #27673, #4557, .T. ) ;
#36729=ORIENTED_EDGE ( 'NONE', *, *, #40798, .T. ) ;
#36764=DIRECTION ( 'NONE',  ( -0.8636456077245080465, 0.5040994586965603652, 0.000000000000000000 ) ) ;
#36847=VERTEX_POINT ( 'NONE', #29862 ) ;
#36875=DIRECTION ( 'NONE',  ( 0.000000000000000000, 0.000000000000000000, -1.000000000000000000 ) ) ;
#36883=CARTESIAN_POINT ( 'NONE',  ( 88.22708560785949317, -3.622631779710408395, -18.64321520033831803 ) ) ;
#36929=CARTESIAN_POINT ( 'NONE',  ( 82.31000308962319423, -13.76004065658516673, -9.893215200338316251 ) ) ;
#36947=VERTEX_POINT ( 'NONE', #43778 ) ;
#36956=ORIENTED_EDGE ( 'NONE', *, *, #4563, .F. ) ;
#36959=CARTESIAN_POINT ( 'NONE',  ( 86.34560043013698305, -9.320000780048239619, -9.893215200338316251 ) ) ;
#37033=CARTESIAN_POINT ( 'NONE',  ( 90.15753105894957287, -11.66076665495339881, -13.24321520033831412 ) ) ;
#37044=FACE_OUTER_BOUND ( 'NONE', #6924, .T. ) ;
#37244=ORIENTED_EDGE ( 'NONE', *, *, #38095, .F. ) ;
#37370=FACE_BOUND ( 'NONE', #16039, .T. ) ;
#37401=VERTEX_POINT ( 'NONE', #35505 ) ;
#37404=VECTOR ( 'NONE', #31725, 1000.000000000000000 ) ;
#37414=EDGE_CURVE ( 'NONE', #27673, #17596, #28088, .T. ) ;
#37436=VERTEX_POINT ( 'NONE', #637 ) ;
#37453=CARTESIAN_POINT ( 'NONE',  ( 92.22433883960545131, -8.119819663282910938, -18.64321520033831803 ) ) ;
#37463=SHAPE_REPRESENTATION_RELATIONSHIP ( 'NONE' , 'NONE' ,  #26250, #34112 ) ;
#37552=EDGE_CURVE ( 'NONE', #33083, #17073, #25717, .T. ) ;
#37584=DIRECTION ( 'NONE',  ( 0.5040994586965589219, 0.8636456077245088236, 0.000000000000000000 ) ) ;
#37632=CARTESIAN_POINT ( 'NONE',  ( 89.16950374942143753, -10.33215483242199717, -14.02354088222794637 ) ) ;
#37653=VECTOR ( 'NONE', #9422, 1000.000000000000000 ) ;
#37659=EDGE_CURVE ( 'NONE', #9906, #19817, #20457, .T. ) ;
#37743=VECTOR ( 'NONE', #40099, 1000.000000000000000 ) ;
#37757=VERTEX_POINT ( 'NONE', #7645 ) ;
#37764=ORIENTED_EDGE ( 'NONE', *, *, #41240, .F. ) ;
#37788=LINE ( 'NONE', #13634, #21893 ) ;
#37803=LINE ( 'NONE', #44894, #19178 ) ;
#37849=CARTESIAN_POINT ( 'NONE',  ( 89.03851648532334195, -10.64689777002964455, -14.14321520033831803 ) ) ;
#37918=PRODUCT_DEFINITION_CONTEXT ( 'detailed design', #23302, 'design' ) ;
#37937=ORIENTED_EDGE ( 'NONE', *, *, #20073, .T. ) ;
#37941=AXIS2_PLACEMENT_3D ( 'NONE', #28502, #29162, #14362 ) ;
#38073=CARTESIAN_POINT ( 'NONE',  ( 89.28219092212185615, -9.933696230371026559, -13.53880969525256184 ) ) ;
#38095=EDGE_CURVE ( 'NONE', #33768, #6720, #18810, .T. ) ;
#38134=DIRECTION ( 'NONE',  ( 0.000000000000000000, 0.000000000000000000, -1.000000000000000000 ) ) ;
#38164=VERTEX_POINT ( 'NONE', #13506 ) ;
#38193=ORIENTED_EDGE ( 'NONE', *, *, #19475, .T. ) ;
#38198=ORIENTED_EDGE ( 'NONE', *, *, #16105, .F. ) ;
#38259=LINE ( 'NONE', #20951, #44436 ) ;
#38299=AXIS2_PLACEMENT_3D ( 'NONE', #18007, #14588, #28506 ) ;
#38324=DIRECTION ( 'NONE',  ( -0.8636456077245090457, 0.5040994586965585889, 0.000000000000000000 ) ) ;
#38357=CARTESIAN_POINT ( 'NONE',  ( 85.45605303719084134, -15.74807682313488222, -13.39321520033831447 ) ) ;
#38409=EDGE_CURVE ( 'NONE', #19235, #12781, #21676, .T. ) ;
#38458=VERTEX_POINT ( 'NONE', #17809 ) ;
#38513=DIRECTION ( 'NONE',  ( 0.000000000000000000, 0.000000000000000000, 1.000000000000000000 ) ) ;
#38519=ORIENTED_EDGE ( 'NONE', *, *, #17306, .T. ) ;
#38611=VERTEX_POINT ( 'NONE', #14386 ) ;
#38640=CARTESIAN_POINT ( 'NONE',  ( 88.22708560785949317, -3.622631779710408395, -18.64321520033831803 ) ) ;
#38710=CARTESIAN_POINT ( 'NONE',  ( 86.39381242489322688, -8.190259192973641689, -8.143215200338314474 ) ) ;
#38722=VECTOR ( 'NONE', #34429, 1000.000000000000000 ) ;
#38732=CYLINDRICAL_SURFACE ( 'NONE', #15558, 0.8999999999999980238 ) ;
#38746=DIRECTION ( 'NONE',  ( 0.000000000000000000, 0.000000000000000000, 1.000000000000000000 ) ) ;
#38748=LINE ( 'NONE', #6862, #1585 ) ;
#38775=VERTEX_POINT ( 'NONE', #23490 ) ;
#38820=ORIENTED_EDGE ( 'NONE', *, *, #40951, .F. ) ;
#38837=VERTEX_POINT ( 'NONE', #33951 ) ;
#38953=CARTESIAN_POINT ( 'NONE',  ( 77.05532149770296257, 0.06670422450934243574, -18.64321520033831803 ) ) ;
#38963=ADVANCED_FACE ( 'NONE', ( #10696 ), #18438, .F. ) ;
#38967=CARTESIAN_POINT ( 'NONE',  ( 88.71490820114844666, -11.16028234076525649, -14.09374590680978123 ) ) ;
#38990=CARTESIAN_POINT ( 'NONE',  ( 85.72471707980444933, -15.28778963902104060, -18.64321520033831803 ) ) ;
#39035=ORIENTED_EDGE ( 'NONE', *, *, #4405, .F. ) ;
#39106=VECTOR ( 'NONE', #20232, 1000.000000000000000 ) ;
#39164=CARTESIAN_POINT ( 'NONE',  ( 74.66232006577804725, -2.500611837642884527, -16.89321520033831447 ) ) ;
#39189=CARTESIAN_POINT ( 'NONE',  ( 75.95778847736481509, -3.256761025687722189, -8.143215200338314474 ) ) ;
#39195=CARTESIAN_POINT ( 'NONE',  ( 88.29631842898217542, -11.60200380960594124, -13.43366796978234845 ) ) ;
#39204=CARTESIAN_POINT ( 'NONE',  ( 73.60369002873177635, -5.846784287000932778, -18.64321520033831803 ) ) ;
#39207=CARTESIAN_POINT ( 'NONE',  ( 86.34560043013698305, -9.320000780048239619, -18.64321520033831803 ) ) ;
#39225=DIRECTION ( 'NONE',  ( 0.5040994586965589219, 0.8636456077245088236, 0.000000000000000000 ) ) ;
#39230=FACE_OUTER_BOUND ( 'NONE', #2013, .T. ) ;
#39244=DIRECTION ( 'NONE',  ( 0.000000000000000000, 0.000000000000000000, 1.000000000000000000 ) ) ;
#39275=ORIENTED_EDGE ( 'NONE', *, *, #25596, .T. ) ;
#39293=CARTESIAN_POINT ( 'NONE',  ( 85.45605303719084134, -15.74807682313488222, -16.89321520033831447 ) ) ;
#39322=EDGE_CURVE ( 'NONE', #32138, #17073, #40758, .T. ) ;
#39403=VECTOR ( 'NONE', #12641, 1000.000000000000114 ) ;
#39428=VECTOR ( 'NONE', #8802, 1000.000000000000000 ) ;
#39443=EDGE_LOOP ( 'NONE', ( #6163, #35495, #44901, #1818 ) ) ;
#39493=VECTOR ( 'NONE', #20697, 1000.000000000000114 ) ;
#39556=DIRECTION ( 'NONE',  ( 0.000000000000000000, 0.000000000000000000, -1.000000000000000000 ) ) ;
#39570=CARTESIAN_POINT ( 'NONE',  ( 86.34560043013698305, -9.320000780048239619, -8.143215200338314474 ) ) ;
#39670=DIRECTION ( 'NONE',  ( 0.000000000000000000, 0.000000000000000000, -1.000000000000000000 ) ) ;
#39790=CARTESIAN_POINT ( 'NONE',  ( 88.22708560785949317, -3.622631779710408395, -18.64321520033831803 ) ) ;
#39793=DIRECTION ( 'NONE',  ( -0.8636456077245092677, 0.5040994586965584778, 0.000000000000000000 ) ) ;
#39840=MECHANICAL_DESIGN_GEOMETRIC_PRESENTATION_REPRESENTATION('',(#7091),#3451);
#39847=CARTESIAN_POINT ( 'NONE',  ( 85.84150097144041069, -10.18364638777274855, -8.143215200338314474 ) ) ;
#39865=CARTESIAN_POINT ( 'NONE',  ( 75.95778847736481509, -3.256761025687722189, -18.64321520033831803 ) ) ;
#39878=CARTESIAN_POINT ( 'NONE',  ( 88.88468749803642766, -10.91782331763674385, -14.14321520033831625 ) ) ;
#39882=CARTESIAN_POINT ( 'NONE',  ( 86.34560043013698305, -9.320000780048239619, -9.893215200338316251 ) ) ;
#39953=CARTESIAN_POINT ( 'NONE',  ( 74.66232006577804725, -2.500611837642884527, -7.993215200338315007 ) ) ;
#40046=CIRCLE ( 'NONE', #28397, 3.000000000000003997 ) ;
#40099=DIRECTION ( 'NONE',  ( 0.000000000000000000, 0.000000000000000000, 1.000000000000000000 ) ) ;
#40116=CARTESIAN_POINT ( 'NONE',  ( 74.66232006577804725, -2.500611837642884527, -7.993215200338315007 ) ) ;
#40147=ORIENTED_EDGE ( 'NONE', *, *, #45087, .T. ) ;
#40151=EDGE_CURVE ( 'NONE', #37757, #38164, #22414, .T. ) ;
#40247=CYLINDRICAL_SURFACE ( 'NONE', #31142, 1.499999999999996225 ) ;
#40278=AXIS2_PLACEMENT_3D ( 'NONE', #41406, #30448, #17226 ) ;
#40290=DIRECTION ( 'NONE',  ( 0.000000000000000000, 0.000000000000000000, -1.000000000000000000 ) ) ;
#40292=DIRECTION ( 'NONE',  ( 0.5040994586965589219, 0.8636456077245088236, 0.000000000000000000 ) ) ;
#40495=CYLINDRICAL_SURFACE ( 'NONE', #11347, 1.499999999999996225 ) ;
#40552=ORIENTED_EDGE ( 'NONE', *, *, #19475, .F. ) ;
#40561=ORIENTED_EDGE ( 'NONE', *, *, #8562, .T. ) ;
#40664=CARTESIAN_POINT ( 'NONE',  ( 85.72471707980444933, -15.28778963902104060, -9.893215200338316251 ) ) ;
#40742=VECTOR ( 'NONE', #35020, 1000.000000000000114 ) ;
#40758=LINE ( 'NONE', #23890, #33963 ) ;
#40793=AXIS2_PLACEMENT_3D ( 'NONE', #11355, #855, #29126 ) ;
#40798=EDGE_CURVE ( 'NONE', #34402, #44995, #19515, .T. ) ;
#40800=LINE ( 'NONE', #1794, #27213 ) ;
#40843=ORIENTED_EDGE ( 'NONE', *, *, #25319, .T. ) ;
#40951=EDGE_CURVE ( 'NONE', #10999, #37436, #11993, .T. ) ;
#41018=CARTESIAN_POINT ( 'NONE',  ( 73.60369002873177635, -5.846784287000932778, -18.64321520033831803 ) ) ;
#41038=CIRCLE ( 'NONE', #6057, 3.000000000000003997 ) ;
#41074=CARTESIAN_POINT ( 'NONE',  ( 89.27809288332949222, -9.952843041749929398, -13.58709681493693644 ) ) ;
#41085=EDGE_LOOP ( 'NONE', ( #13690, #4992, #26066, #17325 ) ) ;
#41090=ORIENTED_EDGE ( 'NONE', *, *, #43156, .F. ) ;
#41111=VERTEX_POINT ( 'NONE', #15635 ) ;
#41240=EDGE_CURVE ( 'NONE', #38837, #38458, #1721, .T. ) ;
#41271=DIRECTION ( 'NONE',  ( 0.5040994586965589219, 0.8636456077245088236, 0.000000000000000000 ) ) ;
#41313=ORIENTED_EDGE ( 'NONE', *, *, #29837, .F. ) ;
#41325=VERTEX_POINT ( 'NONE', #33390 ) ;
#41342=ADVANCED_FACE ( 'NONE', ( #37044 ), #40495, .T. ) ;
#41371=ORIENTED_EDGE ( 'NONE', *, *, #10840, .F. ) ;
#41375=FACE_OUTER_BOUND ( 'NONE', #4205, .T. ) ;
#41378=VERTEX_POINT ( 'NONE', #9940 ) ;
#41379=ADVANCED_FACE ( 'NONE', ( #20649 ), #13802, .F. ) ;
#41385=DIRECTION ( 'NONE',  ( -0.8636456077245080465, 0.5040994586965603652, 0.000000000000000000 ) ) ;
#41406=CARTESIAN_POINT ( 'NONE',  ( 86.34560043013698305, -9.320000780048239619, -18.64321520033831803 ) ) ;
#41446=ORIENTED_EDGE ( 'NONE', *, *, #3382, .F. ) ;
#41542=CIRCLE ( 'NONE', #2190, 3.000000000000003997 ) ;
#41564=AXIS2_PLACEMENT_3D ( 'NONE', #29827, #36875, #19566 ) ;
#41605=AXIS2_PLACEMENT_3D ( 'NONE', #43869, #26766, #10726 ) ;
#41655=DIRECTION ( 'NONE',  ( -0.3135808629537518155, -0.9495615000563051300, -0.000000000000000000 ) ) ;
#41656=AXIS2_PLACEMENT_3D ( 'NONE', #39207, #4545, #28956 ) ;
#41734=CARTESIAN_POINT ( 'NONE',  ( 89.28805143673710631, -9.905285955282378652, -13.44403546754823786 ) ) ;
#41781=AXIS2_PLACEMENT_3D ( 'NONE', #19233, #33116, #36764 ) ;
#41837=ORIENTED_EDGE ( 'NONE', *, *, #30909, .F. ) ;
#41880=DIRECTION ( 'NONE',  ( -0.5040994586965557023, -0.8636456077245108220, 0.000000000000000000 ) ) ;
#41917=ORIENTED_EDGE ( 'NONE', *, *, #25319, .F. ) ;
#41953=CARTESIAN_POINT ( 'NONE',  ( 85.83930302032702286, -9.140269361470597431, -14.14321520033831625 ) ) ;
#41965=CYLINDRICAL_SURFACE ( 'NONE', #32474, 3.000000000000003997 ) ;
#41967=ORIENTED_EDGE ( 'NONE', *, *, #35055, .T. ) ;
#42030=EDGE_CURVE ( 'NONE', #15033, #6780, #12097, .T. ) ;
#42185=CARTESIAN_POINT ( 'NONE',  ( 0.000000000000000000, 0.000000000000000000, 0.000000000000000000 ) ) ;
#42215=DIRECTION ( 'NONE',  ( 0.000000000000000000, 0.000000000000000000, -1.000000000000000000 ) ) ;
#42339=EDGE_CURVE ( 'NONE', #523, #22660, #6688, .T. ) ;
#42500=CARTESIAN_POINT ( 'NONE',  ( 91.23658249893594530, -5.844616714554617509, -9.893215200338316251 ) ) ;
#42601=EDGE_CURVE ( 'NONE', #16972, #16620, #33989, .T. ) ;
#42630=CARTESIAN_POINT ( 'NONE',  ( 88.28425963449632263, -11.60945497031996787, -13.24321520033830879 ) ) ;
#42636=FACE_OUTER_BOUND ( 'NONE', #10134, .T. ) ;
#42693=ORIENTED_EDGE ( 'NONE', *, *, #203, .T. ) ;
#42762=AXIS2_PLACEMENT_3D ( 'NONE', #36284, #22389, #43141 ) ;
#42840=CARTESIAN_POINT ( 'NONE',  ( 74.66232006577804725, -2.500611837642884527, -18.79321520033831661 ) ) ;
#42849=FACE_OUTER_BOUND ( 'NONE', #29458, .T. ) ;
#42854=CARTESIAN_POINT ( 'NONE',  ( 88.66111334384352460, -11.22778238082202407, -14.05973504337623581 ) ) ;
#42871=DIRECTION ( 'NONE',  ( 0.000000000000000000, 0.000000000000000000, -1.000000000000000000 ) ) ;
#42873=ORIENTED_EDGE ( 'NONE', *, *, #40798, .F. ) ;
#42875=LINE ( 'NONE', #38990, #19646 ) ;
#42886=CARTESIAN_POINT ( 'NONE',  ( 77.25325688895158294, -4.012910213732562070, -9.893215200338316251 ) ) ;
#42896=ORIENTED_EDGE ( 'NONE', *, *, #38409, .F. ) ;
#42916=ORIENTED_EDGE ( 'NONE', *, *, #15908, .T. ) ;
#42926=DIRECTION ( 'NONE',  ( 0.000000000000000000, 0.000000000000000000, -1.000000000000000000 ) ) ;
#42935=FACE_OUTER_BOUND ( 'NONE', #21685, .T. ) ;
#42975=EDGE_CURVE ( 'NONE', #9906, #523, #6337, .T. ) ;
#43025=VECTOR ( 'NONE', #31153, 1000.000000000000000 ) ;
#43039=AXIS2_PLACEMENT_3D ( 'NONE', #39865, #9080, #35976 ) ;
#43106=PLANE ( 'NONE',  #21133 ) ;
#43141=DIRECTION ( 'NONE',  ( 0.8636456077245089347, -0.5040994586965589219, 0.000000000000000000 ) ) ;
#43156=EDGE_CURVE ( 'NONE', #41325, #10999, #25251, .T. ) ;
#43236=CIRCLE ( 'NONE', #41781, 1.499999999999996225 ) ;
#43243=LINE ( 'NONE', #36377, #39428 ) ;
#43252=VECTOR ( 'NONE', #35449, 1000.000000000000000 ) ;
#43263=CLOSED_SHELL ( 'NONE', ( #21205, #8887, #41379, #38963, #4823, #25571, #17899, #30115, #32588, #6075, #36251, #43665, #2894, #11074, #23822, #4515, #15325, #34270, #5025, #29852, #9130, #13376, #15628, #8833, #24313, #31156, #44902, #3002, #41342, #6885 ) ) ;
#43310=B_SPLINE_CURVE_WITH_KNOTS ( 'NONE', 3,
 ( #7066, #10061, #27152, #41734, #2971, #20090, #38073, #33976, #10498, #17121, #41074, #3636, #31010, #24620, #6170, #34416, #23964, #6851, #17554, #37632, #27605, #44483, #31448, #20758, #218, #20313, #14131, #20536, #37849, #28047 ),
 .UNSPECIFIED., .F., .F.,
 ( 4, 2, 2, 1, 1, 2, 2, 2, 2, 2, 2, 2, 1, 1, 2, 2, 4 ),
 ( 0.000000000000000000, 0.1249999999999235056, 0.1874999999998855915, 0.2187499999998666345, 0.2343749999998555322, 0.2421874999998526456, 0.2499999999998497868, 0.3749999999999040212, 0.4374999999999267808, 0.4999999999999494849, 0.6249999999999925615, 0.6875000000000155431, 0.7187500000000270894, 0.7343750000000252021, 0.7421875000000229816, 0.7500000000000207612, 1.000000000000000000 ),
 .UNSPECIFIED. ) ;
#43318=VERTEX_POINT ( 'NONE', #3709 ) ;
#43327=DIRECTION ( 'NONE',  ( -0.7400066460894876297, 0.6725995567522979890, 0.000000000000000000 ) ) ;
#43336=ORIENTED_EDGE ( 'NONE', *, *, #28759, .T. ) ;
#43343=VERTEX_POINT ( 'NONE', #45011 ) ;
#43353=ORIENTED_EDGE ( 'NONE', *, *, #7730, .T. ) ;
#43367=FACE_BOUND ( 'NONE', #23129, .T. ) ;
#43372=ORIENTED_EDGE ( 'NONE', *, *, #3382, .T. ) ;
#43504=VECTOR ( 'NONE', #14905, 1000.000000000000000 ) ;
#43538=DIRECTION ( 'NONE',  ( 0.000000000000000000, 0.000000000000000000, -1.000000000000000000 ) ) ;
#43542=DIRECTION ( 'NONE',  ( 0.5040994586965589219, 0.8636456077245089347, 0.000000000000000000 ) ) ;
#43552=FACE_OUTER_BOUND ( 'NONE', #33585, .T. ) ;
#43645=DIRECTION ( 'NONE',  ( -0.8636456077245080465, 0.5040994586965603652, 0.000000000000000000 ) ) ;
#43665=ADVANCED_FACE ( 'NONE', ( #43367, #15324 ), #22611, .F. ) ;
#43679=DIRECTION ( 'NONE',  ( 0.000000000000000000, 0.000000000000000000, -1.000000000000000000 ) ) ;
#43699=SHAPE_DEFINITION_REPRESENTATION ( #831, #26250 ) ;
#43740=FACE_OUTER_BOUND ( 'NONE', #41085, .T. ) ;
#43741=DIRECTION ( 'NONE',  ( 0.8636456077245086016, -0.5040994586965593660, 0.000000000000000000 ) ) ;
#43767=EDGE_LOOP ( 'NONE', ( #33692, #34386, #18966, #41837 ) ) ;
#43778=CARTESIAN_POINT ( 'NONE',  ( 82.31000308962319423, -13.76004065658516673, -9.893215200338316251 ) ) ;
#43819=ORIENTED_EDGE ( 'NONE', *, *, #9602, .F. ) ;
#43869=CARTESIAN_POINT ( 'NONE',  ( 86.34560043013698305, -9.320000780048239619, -18.64321520033831803 ) ) ;
#43875=AXIS2_PLACEMENT_3D ( 'NONE', #19821, #8881, #43542 ) ;
#43972=ORIENTED_EDGE ( 'NONE', *, *, #32280, .F. ) ;
#43978=DIRECTION ( 'NONE',  ( -0.3135808629537518155, -0.9495615000563051300, -0.000000000000000000 ) ) ;
#44018=CIRCLE ( 'NONE', #22166, 3.000000000000003997 ) ;
#44077=CARTESIAN_POINT ( 'NONE',  ( 82.31000308962319423, -13.76004065658516673, -18.64321520033831803 ) ) ;
#44151=LINE ( 'NONE', #6046, #13891 ) ;
#44182=CARTESIAN_POINT ( 'NONE',  ( 90.71204046351577688, -10.71075648645643774, -8.143215200338314474 ) ) ;
#44381=VERTEX_POINT ( 'NONE', #2828 ) ;
#44387=ORIENTED_EDGE ( 'NONE', *, *, #22776, .T. ) ;
#44436=VECTOR ( 'NONE', #41271, 1000.000000000000000 ) ;
#44483=CARTESIAN_POINT ( 'NONE',  ( 89.15006894847832086, -10.38507692083869038, -14.05253605978568743 ) ) ;
#44507=VERTEX_POINT ( 'NONE', #44796 ) ;
#44531=EDGE_CURVE ( 'NONE', #41378, #15181, #17284, .T. ) ;
#44729=AXIS2_PLACEMENT_3D ( 'NONE', #26334, #35679, #4453 ) ;
#44796=CARTESIAN_POINT ( 'NONE',  ( 83.75466360696344736, -7.807702403958562520, -18.64321520033831803 ) ) ;
#44799=CARTESIAN_POINT ( 'NONE',  ( 92.22433883960545131, -8.119819663282910938, -8.143215200338314474 ) ) ;
#44842=ORIENTED_EDGE ( 'NONE', *, *, #37659, .T. ) ;
#44856=AXIS2_PLACEMENT_3D ( 'NONE', #13361, #23853, #17665 ) ;
#44894=CARTESIAN_POINT ( 'NONE',  ( 90.20794100481921873, -11.57440209418094668, -8.143215200338314474 ) ) ;
#44901=ORIENTED_EDGE ( 'NONE', *, *, #35895, .T. ) ;
#44902=ADVANCED_FACE ( 'NONE', ( #42636 ), #41965, .F. ) ;
#44911=CARTESIAN_POINT ( 'NONE',  ( 75.95778847736481509, -3.256761025687722189, -16.89321520033831447 ) ) ;
#44918=AXIS2_PLACEMENT_3D ( 'NONE', #25652, #39556, #43645 ) ;
#44948=DIRECTION ( 'NONE',  ( -0.8636456077245092677, 0.5040994586965584778, 0.000000000000000000 ) ) ;
#44964=ORIENTED_EDGE ( 'NONE', *, *, #29837, .T. ) ;
#44995=VERTEX_POINT ( 'NONE', #1790 ) ;
#44996=CARTESIAN_POINT ( 'NONE',  ( 77.25325688895158294, -4.012910213732562070, -7.993215200338315007 ) ) ;
#45011=CARTESIAN_POINT ( 'NONE',  ( 90.25835095068887881, -11.48803753340850164, -14.14321520033831625 ) ) ;
#45083=DIRECTION ( 'NONE',  ( -0.8636456077245092677, 0.5040994586965584778, 0.000000000000000000 ) ) ;
#45087=EDGE_CURVE ( 'NONE', #6720, #19850, #22547, .T. ) ;
#45163=COLOUR_RGB('Light Blue',0.38,0.62,0.78);
#45164=FILL_AREA_STYLE_COLOUR('',#45163);
#45165=FILL_AREA_STYLE('',(#45164));
#45166=SURFACE_STYLE_FILL_AREA(#45165);
#45167=SURFACE_SIDE_STYLE('',(#45166));
#45168=SURFACE_STYLE_USAGE(.BOTH.,#45167);
#45169=PRESENTATION_STYLE_ASSIGNMENT((#45168));
ENDSEC;
END-ISO-10303-21;
